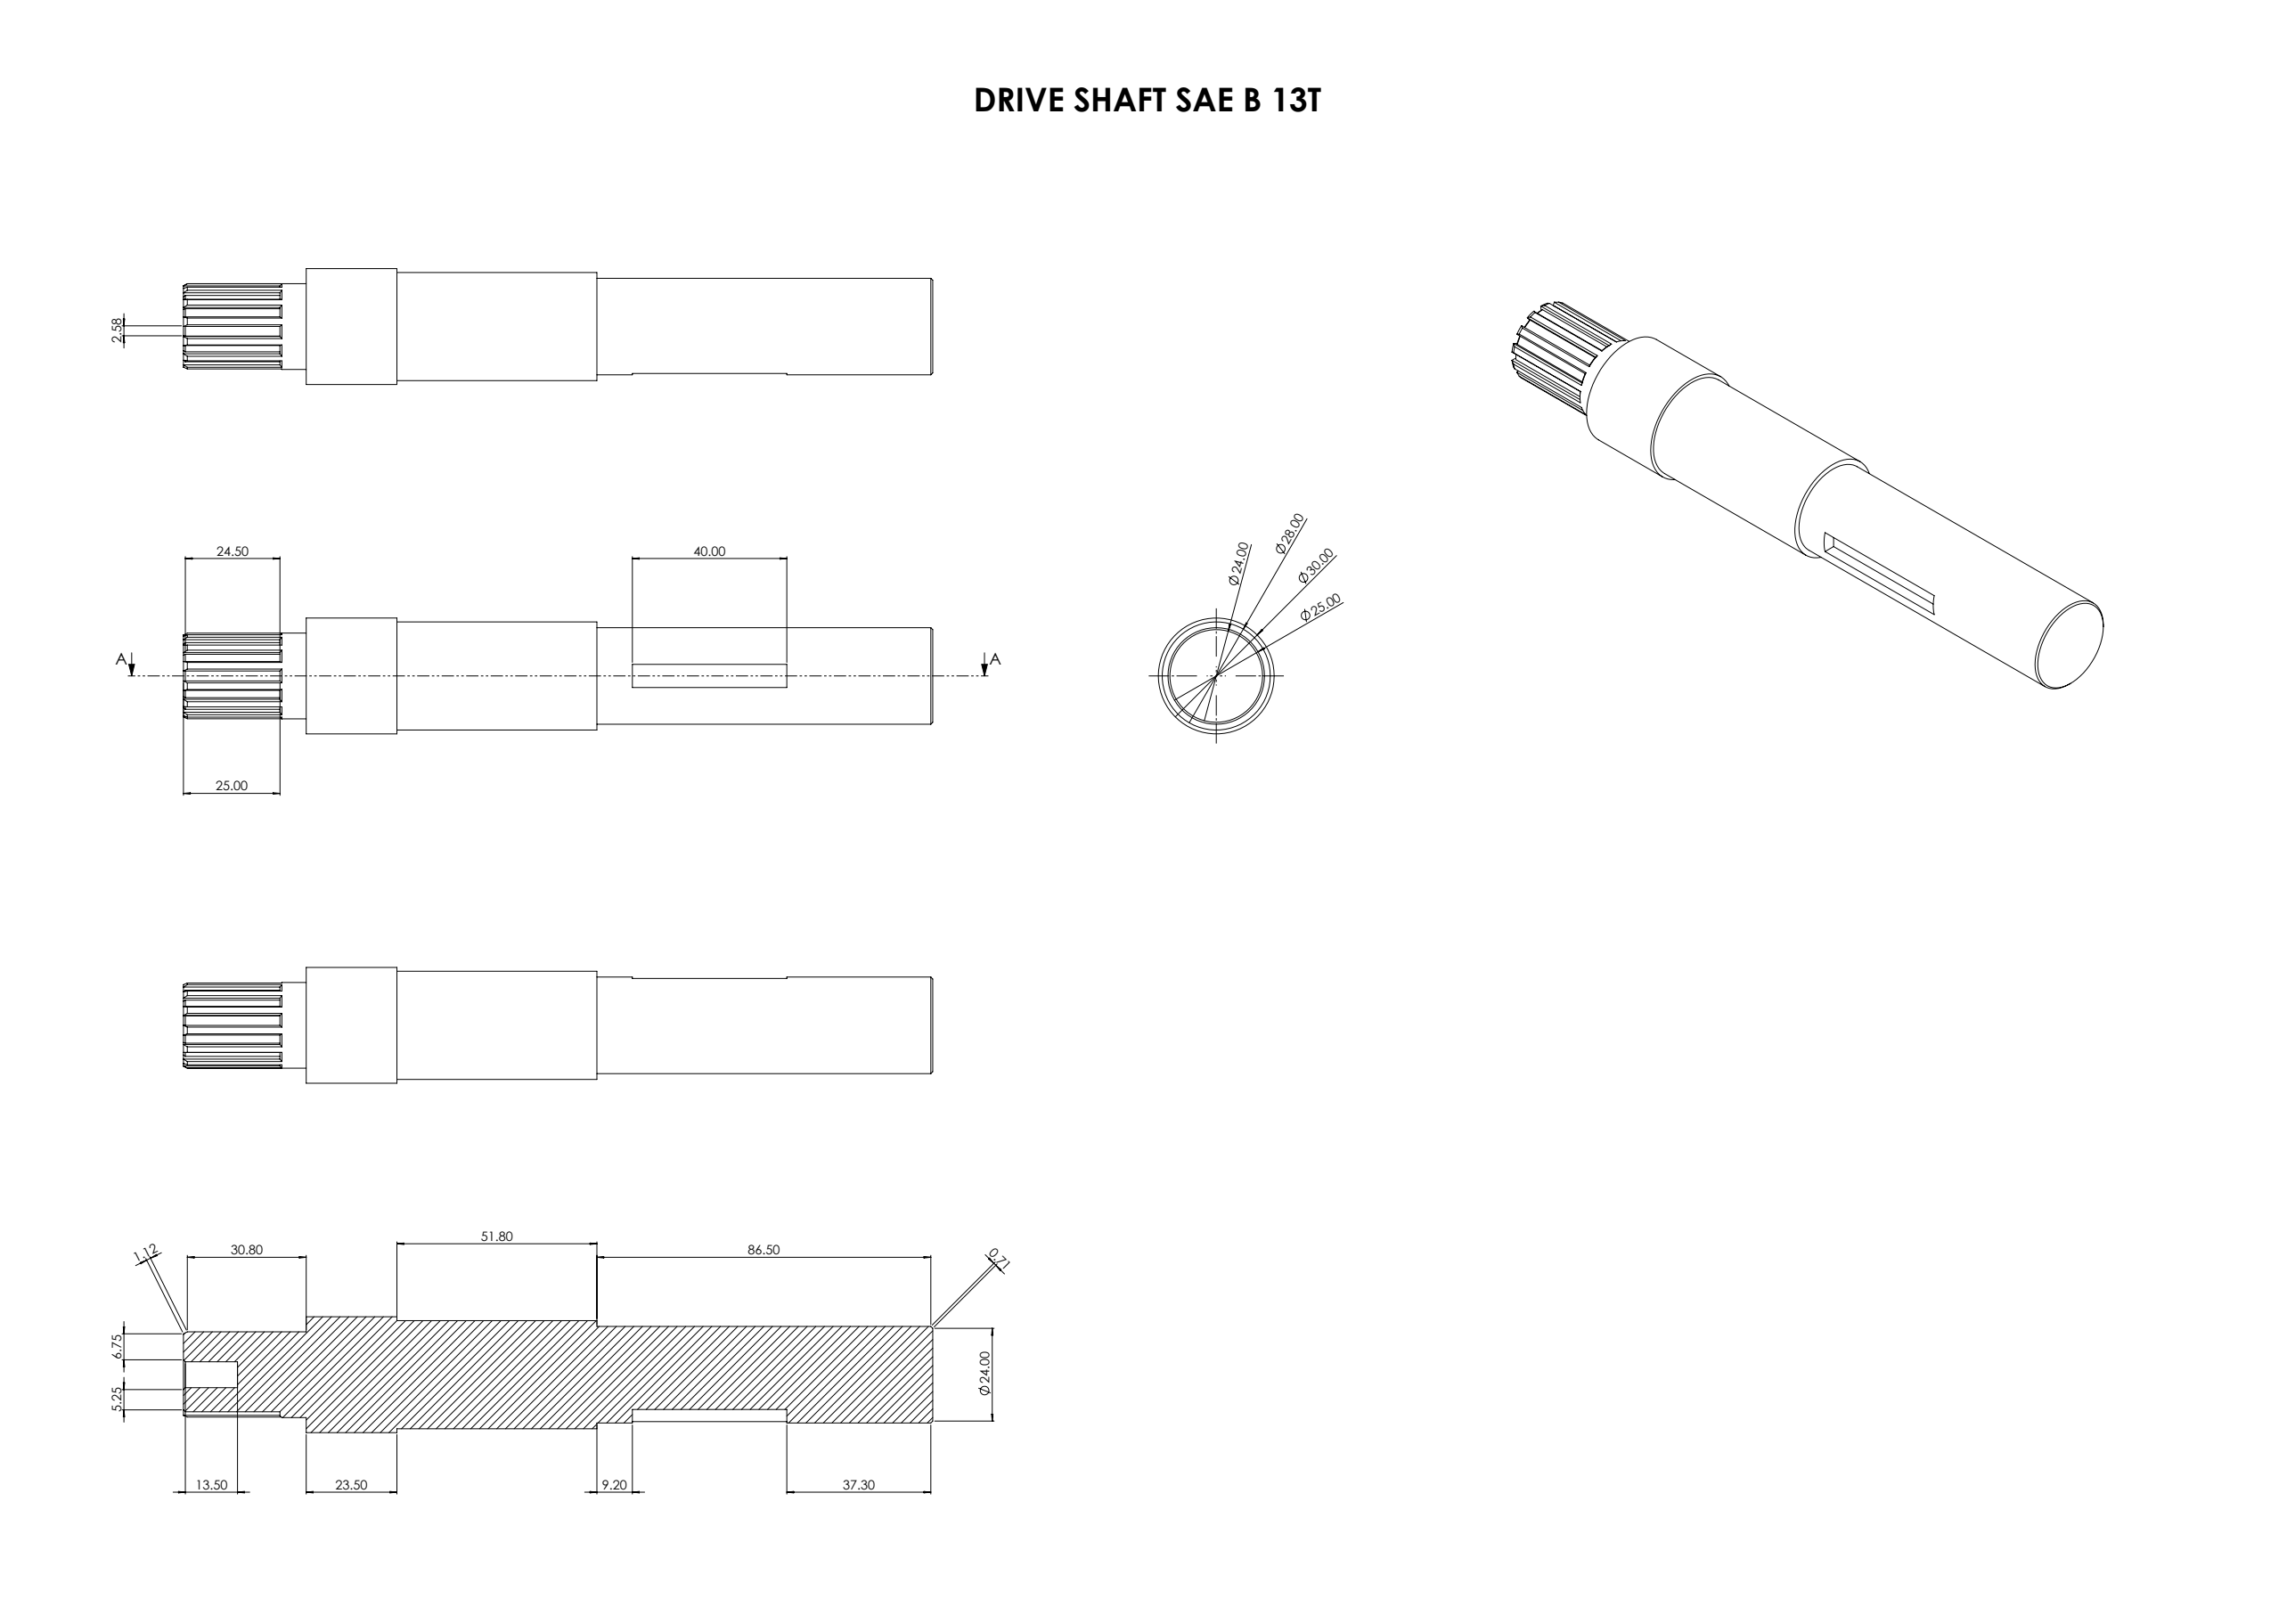
ISO-10303-21;
HEADER;
/* Generated by software containing ST-Developer
 * from STEP Tools, Inc. (www.steptools.com) 
 */

FILE_DESCRIPTION(
/* description */ (''),
/* implementation_level */ '2;1');

FILE_NAME(
/* name */ '09_Drive_Shaft_SAE_B_13T.step',
/* time_stamp */ '2026-10-26T07:49:00-07:00',
/* author */ (''),
/* organization */ (''),
/* preprocessor_version */ 'ST-DEVELOPER v20.2',
/* originating_system */ 'Autodesk Translation Framework v15.15.0.0',
/* authorisation */ '');

FILE_SCHEMA (('AUTOMOTIVE_DESIGN { 1 0 10303 214 3 1 1 }'));
ENDSEC;

DATA;
#10=MECHANICAL_DESIGN_GEOMETRIC_PRESENTATION_REPRESENTATION('',(#182),#38507);
#152=SHAPE_REPRESENTATION_RELATIONSHIP('SRR','None',#38580,#167);
#167=ADVANCED_BREP_SHAPE_REPRESENTATION('',(#197),#38497);
#182=STYLED_ITEM('',(#38720),#197);
#197=MANIFOLD_SOLID_BREP('Body1',#15076);
#338=(
BOUNDED_CURVE()
B_SPLINE_CURVE(2,(#25747,#25748,#25749),.UNSPECIFIED.,.F.,.F.)
B_SPLINE_CURVE_WITH_KNOTS((3,3),(0.00089915875038223,0.119861415155793),
 .UNSPECIFIED.)
CURVE()
GEOMETRIC_REPRESENTATION_ITEM()
RATIONAL_B_SPLINE_CURVE((1.00000690885838,1.00046048906391,1.))
REPRESENTATION_ITEM('')
);
#339=(
BOUNDED_CURVE()
B_SPLINE_CURVE(2,(#25761,#25762,#25763),.UNSPECIFIED.,.F.,.F.)
B_SPLINE_CURVE_WITH_KNOTS((3,3),(0.,0.118962256406331),.UNSPECIFIED.)
CURVE()
GEOMETRIC_REPRESENTATION_ITEM()
RATIONAL_B_SPLINE_CURVE((1.,1.00046048906569,1.0000069088584))
REPRESENTATION_ITEM('')
);
#340=(
BOUNDED_CURVE()
B_SPLINE_CURVE(2,(#25773,#25774,#25775),.UNSPECIFIED.,.F.,.F.)
B_SPLINE_CURVE_WITH_KNOTS((3,3),(-47.8696729569845,-47.8687190848821),
 .UNSPECIFIED.)
CURVE()
GEOMETRIC_REPRESENTATION_ITEM()
RATIONAL_B_SPLINE_CURVE((15.2054806811783,15.2077824060813,15.2100840336135))
REPRESENTATION_ITEM('')
);
#341=(
BOUNDED_CURVE()
B_SPLINE_CURVE(2,(#25778,#25779,#25780),.UNSPECIFIED.,.F.,.F.)
B_SPLINE_CURVE_WITH_KNOTS((3,3),(-2.77393487400909,-2.77298100190668),
 .UNSPECIFIED.)
CURVE()
GEOMETRIC_REPRESENTATION_ITEM()
RATIONAL_B_SPLINE_CURVE((15.2100840336134,15.2077824060812,15.2054806811782))
REPRESENTATION_ITEM('')
);
#342=(
BOUNDED_CURVE()
B_SPLINE_CURVE(2,(#25790,#25791,#25792),.UNSPECIFIED.,.F.,.F.)
B_SPLINE_CURVE_WITH_KNOTS((3,3),(0.111140514111159,0.111966209987666),
 .UNSPECIFIED.)
CURVE()
GEOMETRIC_REPRESENTATION_ITEM()
RATIONAL_B_SPLINE_CURVE((1.00000394455129,1.00000198692827,1.))
REPRESENTATION_ITEM('')
);
#343=(
BOUNDED_CURVE()
B_SPLINE_CURVE(2,(#25799,#25800,#25801),.UNSPECIFIED.,.F.,.F.)
B_SPLINE_CURVE_WITH_KNOTS((3,3),(0.,0.000825695876467816),.UNSPECIFIED.)
CURVE()
GEOMETRIC_REPRESENTATION_ITEM()
RATIONAL_B_SPLINE_CURVE((1.,1.00000198692868,1.00000394455211))
REPRESENTATION_ITEM('')
);
#344=(
BOUNDED_CURVE()
B_SPLINE_CURVE(2,(#25812,#25813,#25814),.UNSPECIFIED.,.F.,.F.)
B_SPLINE_CURVE_WITH_KNOTS((3,3),(0.000899158750379295,0.119861415155793),
 .UNSPECIFIED.)
CURVE()
GEOMETRIC_REPRESENTATION_ITEM()
RATIONAL_B_SPLINE_CURVE((1.00000690885842,1.00046048906656,1.))
REPRESENTATION_ITEM('')
);
#345=(
BOUNDED_CURVE()
B_SPLINE_CURVE(2,(#25826,#25827,#25828),.UNSPECIFIED.,.F.,.F.)
B_SPLINE_CURVE_WITH_KNOTS((3,3),(0.,0.11896225640633),.UNSPECIFIED.)
CURVE()
GEOMETRIC_REPRESENTATION_ITEM()
RATIONAL_B_SPLINE_CURVE((1.,1.00046048906395,1.00000690885837))
REPRESENTATION_ITEM('')
);
#346=(
BOUNDED_CURVE()
B_SPLINE_CURVE(2,(#25838,#25839,#25840),.UNSPECIFIED.,.F.,.F.)
B_SPLINE_CURVE_WITH_KNOTS((3,3),(-47.8696729569843,-47.8687190848819),
 .UNSPECIFIED.)
CURVE()
GEOMETRIC_REPRESENTATION_ITEM()
RATIONAL_B_SPLINE_CURVE((15.2054806811781,15.2077824060811,15.2100840336132))
REPRESENTATION_ITEM('')
);
#347=(
BOUNDED_CURVE()
B_SPLINE_CURVE(2,(#25843,#25844,#25845),.UNSPECIFIED.,.F.,.F.)
B_SPLINE_CURVE_WITH_KNOTS((3,3),(-2.77393487400938,-2.77298100190697),
 .UNSPECIFIED.)
CURVE()
GEOMETRIC_REPRESENTATION_ITEM()
RATIONAL_B_SPLINE_CURVE((15.2100840336132,15.2077824060811,15.2054806811781))
REPRESENTATION_ITEM('')
);
#348=(
BOUNDED_CURVE()
B_SPLINE_CURVE(2,(#25855,#25856,#25857),.UNSPECIFIED.,.F.,.F.)
B_SPLINE_CURVE_WITH_KNOTS((3,3),(0.111140514109634,0.111966209987666),
 .UNSPECIFIED.)
CURVE()
GEOMETRIC_REPRESENTATION_ITEM()
RATIONAL_B_SPLINE_CURVE((1.00000394455479,1.00000198693003,1.))
REPRESENTATION_ITEM('')
);
#349=(
BOUNDED_CURVE()
B_SPLINE_CURVE(2,(#25864,#25865,#25866),.UNSPECIFIED.,.F.,.F.)
B_SPLINE_CURVE_WITH_KNOTS((3,3),(0.,0.000825695875370319),.UNSPECIFIED.)
CURVE()
GEOMETRIC_REPRESENTATION_ITEM()
RATIONAL_B_SPLINE_CURVE((1.,1.00000198692765,1.00000394455006))
REPRESENTATION_ITEM('')
);
#350=(
BOUNDED_CURVE()
B_SPLINE_CURVE(2,(#25877,#25878,#25879),.UNSPECIFIED.,.F.,.F.)
B_SPLINE_CURVE_WITH_KNOTS((3,3),(0.000899158750382334,0.119861415155793),
 .UNSPECIFIED.)
CURVE()
GEOMETRIC_REPRESENTATION_ITEM()
RATIONAL_B_SPLINE_CURVE((1.00000690885837,1.00046048906313,1.))
REPRESENTATION_ITEM('')
);
#351=(
BOUNDED_CURVE()
B_SPLINE_CURVE(2,(#25891,#25892,#25893),.UNSPECIFIED.,.F.,.F.)
B_SPLINE_CURVE_WITH_KNOTS((3,3),(0.,0.11896225640633),.UNSPECIFIED.)
CURVE()
GEOMETRIC_REPRESENTATION_ITEM()
RATIONAL_B_SPLINE_CURVE((1.,1.00046048906413,1.00000690885838))
REPRESENTATION_ITEM('')
);
#352=(
BOUNDED_CURVE()
B_SPLINE_CURVE(2,(#25903,#25904,#25905),.UNSPECIFIED.,.F.,.F.)
B_SPLINE_CURVE_WITH_KNOTS((3,3),(-47.8696729569845,-47.8687190848821),
 .UNSPECIFIED.)
CURVE()
GEOMETRIC_REPRESENTATION_ITEM()
RATIONAL_B_SPLINE_CURVE((15.2054806811782,15.2077824060812,15.2100840336134))
REPRESENTATION_ITEM('')
);
#353=(
BOUNDED_CURVE()
B_SPLINE_CURVE(2,(#25908,#25909,#25910),.UNSPECIFIED.,.F.,.F.)
B_SPLINE_CURVE_WITH_KNOTS((3,3),(-2.77393487400914,-2.77298100190673),
 .UNSPECIFIED.)
CURVE()
GEOMETRIC_REPRESENTATION_ITEM()
RATIONAL_B_SPLINE_CURVE((15.2100840336134,15.2077824060812,15.2054806811782))
REPRESENTATION_ITEM('')
);
#354=(
BOUNDED_CURVE()
B_SPLINE_CURVE(2,(#25920,#25921,#25922),.UNSPECIFIED.,.F.,.F.)
B_SPLINE_CURVE_WITH_KNOTS((3,3),(0.111140514110888,0.111966209987666),
 .UNSPECIFIED.)
CURVE()
GEOMETRIC_REPRESENTATION_ITEM()
RATIONAL_B_SPLINE_CURVE((1.000003944553,1.00000198692913,1.))
REPRESENTATION_ITEM('')
);
#355=(
BOUNDED_CURVE()
B_SPLINE_CURVE(2,(#25929,#25930,#25931),.UNSPECIFIED.,.F.,.F.)
B_SPLINE_CURVE_WITH_KNOTS((3,3),(0.,0.000825695876921701),.UNSPECIFIED.)
CURVE()
GEOMETRIC_REPRESENTATION_ITEM()
RATIONAL_B_SPLINE_CURVE((1.,1.0000019869287,1.00000394455216))
REPRESENTATION_ITEM('')
);
#356=(
BOUNDED_CURVE()
B_SPLINE_CURVE(2,(#25942,#25943,#25944),.UNSPECIFIED.,.F.,.F.)
B_SPLINE_CURVE_WITH_KNOTS((3,3),(0.000899158750381089,0.119861415155793),
 .UNSPECIFIED.)
CURVE()
GEOMETRIC_REPRESENTATION_ITEM()
RATIONAL_B_SPLINE_CURVE((1.00000690885838,1.00046048906409,1.))
REPRESENTATION_ITEM('')
);
#357=(
BOUNDED_CURVE()
B_SPLINE_CURVE(2,(#25956,#25957,#25958),.UNSPECIFIED.,.F.,.F.)
B_SPLINE_CURVE_WITH_KNOTS((3,3),(0.,0.118962256406332),.UNSPECIFIED.)
CURVE()
GEOMETRIC_REPRESENTATION_ITEM()
RATIONAL_B_SPLINE_CURVE((1.,1.00046048906654,1.00000690885841))
REPRESENTATION_ITEM('')
);
#358=(
BOUNDED_CURVE()
B_SPLINE_CURVE(2,(#25968,#25969,#25970),.UNSPECIFIED.,.F.,.F.)
B_SPLINE_CURVE_WITH_KNOTS((3,3),(-47.8696729569844,-47.868719084882),
 .UNSPECIFIED.)
CURVE()
GEOMETRIC_REPRESENTATION_ITEM()
RATIONAL_B_SPLINE_CURVE((15.2054806811782,15.2077824060812,15.2100840336134))
REPRESENTATION_ITEM('')
);
#359=(
BOUNDED_CURVE()
B_SPLINE_CURVE(2,(#25973,#25974,#25975),.UNSPECIFIED.,.F.,.F.)
B_SPLINE_CURVE_WITH_KNOTS((3,3),(-2.77393487400941,-2.772981001907),
 .UNSPECIFIED.)
CURVE()
GEOMETRIC_REPRESENTATION_ITEM()
RATIONAL_B_SPLINE_CURVE((15.2100840336131,15.207782406081,15.205480681178))
REPRESENTATION_ITEM('')
);
#360=(
BOUNDED_CURVE()
B_SPLINE_CURVE(2,(#25985,#25986,#25987),.UNSPECIFIED.,.F.,.F.)
B_SPLINE_CURVE_WITH_KNOTS((3,3),(0.111140514110977,0.111966209987666),
 .UNSPECIFIED.)
CURVE()
GEOMETRIC_REPRESENTATION_ITEM()
RATIONAL_B_SPLINE_CURVE((1.00000394455159,1.00000198692842,1.))
REPRESENTATION_ITEM('')
);
#361=(
BOUNDED_CURVE()
B_SPLINE_CURVE(2,(#25994,#25995,#25996),.UNSPECIFIED.,.F.,.F.)
B_SPLINE_CURVE_WITH_KNOTS((3,3),(0.,0.000825695874631881),.UNSPECIFIED.)
CURVE()
GEOMETRIC_REPRESENTATION_ITEM()
RATIONAL_B_SPLINE_CURVE((1.,1.00000198692687,1.00000394454852))
REPRESENTATION_ITEM('')
);
#362=(
BOUNDED_CURVE()
B_SPLINE_CURVE(2,(#26005,#26006,#26007),.UNSPECIFIED.,.F.,.F.)
B_SPLINE_CURVE_WITH_KNOTS((3,3),(0.000899158750383316,0.119861415155793),
 .UNSPECIFIED.)
CURVE()
GEOMETRIC_REPRESENTATION_ITEM()
RATIONAL_B_SPLINE_CURVE((1.00000690885837,1.00046048906313,1.))
REPRESENTATION_ITEM('')
);
#363=(
BOUNDED_CURVE()
B_SPLINE_CURVE(2,(#26011,#26012,#26013),.UNSPECIFIED.,.F.,.F.)
B_SPLINE_CURVE_WITH_KNOTS((3,3),(1.83887863060053,1.88690815084928),
 .UNSPECIFIED.)
CURVE()
GEOMETRIC_REPRESENTATION_ITEM()
RATIONAL_B_SPLINE_CURVE((1.02805437145288,1.01439356064084,1.))
REPRESENTATION_ITEM('')
);
#364=(
BOUNDED_CURVE()
B_SPLINE_CURVE(2,(#26017,#26018,#26019),.UNSPECIFIED.,.F.,.F.)
B_SPLINE_CURVE_WITH_KNOTS((3,3),(0.0704444719086716,0.0709678248042913),
 .UNSPECIFIED.)
CURVE()
GEOMETRIC_REPRESENTATION_ITEM()
RATIONAL_B_SPLINE_CURVE((1.00000394455158,1.00000198692841,1.))
REPRESENTATION_ITEM('')
);
#365=(
BOUNDED_CURVE()
B_SPLINE_CURVE(2,(#26028,#26029,#26030),.UNSPECIFIED.,.F.,.F.)
B_SPLINE_CURVE_WITH_KNOTS((3,3),(0.111140514109306,0.111966209987666),
 .UNSPECIFIED.)
CURVE()
GEOMETRIC_REPRESENTATION_ITEM()
RATIONAL_B_SPLINE_CURVE((1.00000394455327,1.00000198692926,1.))
REPRESENTATION_ITEM('')
);
#366=(
BOUNDED_CURVE()
B_SPLINE_CURVE(2,(#26036,#26037,#26038),.UNSPECIFIED.,.F.,.F.)
B_SPLINE_CURVE_WITH_KNOTS((3,3),(0.,0.118962256406332),.UNSPECIFIED.)
CURVE()
GEOMETRIC_REPRESENTATION_ITEM()
RATIONAL_B_SPLINE_CURVE((1.,1.00046048906504,1.00000690885839))
REPRESENTATION_ITEM('')
);
#367=(
BOUNDED_CURVE()
B_SPLINE_CURVE(2,(#26049,#26050,#26051),.UNSPECIFIED.,.F.,.F.)
B_SPLINE_CURVE_WITH_KNOTS((3,3),(-47.8696729569846,-47.8687190848822),
 .UNSPECIFIED.)
CURVE()
GEOMETRIC_REPRESENTATION_ITEM()
RATIONAL_B_SPLINE_CURVE((15.2054806811784,15.2077824060813,15.2100840336135))
REPRESENTATION_ITEM('')
);
#368=(
BOUNDED_CURVE()
B_SPLINE_CURVE(2,(#26054,#26055,#26056),.UNSPECIFIED.,.F.,.F.)
B_SPLINE_CURVE_WITH_KNOTS((3,3),(0.,0.000825695876215709),.UNSPECIFIED.)
CURVE()
GEOMETRIC_REPRESENTATION_ITEM()
RATIONAL_B_SPLINE_CURVE((1.,1.00000198692775,1.00000394455027))
REPRESENTATION_ITEM('')
);
#369=(
BOUNDED_CURVE()
B_SPLINE_CURVE(2,(#26068,#26069,#26070),.UNSPECIFIED.,.F.,.F.)
B_SPLINE_CURVE_WITH_KNOTS((3,3),(0.000899158750381245,0.119861415155792),
 .UNSPECIFIED.)
CURVE()
GEOMETRIC_REPRESENTATION_ITEM()
RATIONAL_B_SPLINE_CURVE((1.00000690885837,1.00046048906334,1.))
REPRESENTATION_ITEM('')
);
#370=(
BOUNDED_CURVE()
B_SPLINE_CURVE(2,(#26072,#26073,#26074),.UNSPECIFIED.,.F.,.F.)
B_SPLINE_CURVE_WITH_KNOTS((3,3),(0.111140514111096,0.111966209987666),
 .UNSPECIFIED.)
CURVE()
GEOMETRIC_REPRESENTATION_ITEM()
RATIONAL_B_SPLINE_CURVE((1.00000394455331,1.00000198692928,1.))
REPRESENTATION_ITEM('')
);
#371=(
BOUNDED_CURVE()
B_SPLINE_CURVE(2,(#26158,#26159,#26160),.UNSPECIFIED.,.F.,.F.)
B_SPLINE_CURVE_WITH_KNOTS((3,3),(0.,0.118962256406332),.UNSPECIFIED.)
CURVE()
GEOMETRIC_REPRESENTATION_ITEM()
RATIONAL_B_SPLINE_CURVE((1.,1.00046048906488,1.00000690885839))
REPRESENTATION_ITEM('')
);
#372=(
BOUNDED_CURVE()
B_SPLINE_CURVE(2,(#26169,#26170,#26171),.UNSPECIFIED.,.F.,.F.)
B_SPLINE_CURVE_WITH_KNOTS((3,3),(-47.8696729569843,-47.8687190848819),
 .UNSPECIFIED.)
CURVE()
GEOMETRIC_REPRESENTATION_ITEM()
RATIONAL_B_SPLINE_CURVE((15.2054806811781,15.2077824060811,15.2100840336132))
REPRESENTATION_ITEM('')
);
#373=(
BOUNDED_CURVE()
B_SPLINE_CURVE(2,(#26174,#26175,#26176),.UNSPECIFIED.,.F.,.F.)
B_SPLINE_CURVE_WITH_KNOTS((3,3),(-2.77393487400923,-2.77298100190682),
 .UNSPECIFIED.)
CURVE()
GEOMETRIC_REPRESENTATION_ITEM()
RATIONAL_B_SPLINE_CURVE((15.2100840336133,15.2077824060812,15.2054806811782))
REPRESENTATION_ITEM('')
);
#374=(
BOUNDED_CURVE()
B_SPLINE_CURVE(2,(#26191,#26192,#26193),.UNSPECIFIED.,.F.,.F.)
B_SPLINE_CURVE_WITH_KNOTS((3,3),(0.,0.0008256958761486),.UNSPECIFIED.)
CURVE()
GEOMETRIC_REPRESENTATION_ITEM()
RATIONAL_B_SPLINE_CURVE((1.,1.00000198692878,1.00000394455231))
REPRESENTATION_ITEM('')
);
#375=(
BOUNDED_CURVE()
B_SPLINE_CURVE(2,(#26203,#26204,#26205),.UNSPECIFIED.,.F.,.F.)
B_SPLINE_CURVE_WITH_KNOTS((3,3),(0.000899158750380169,0.119861415155792),
 .UNSPECIFIED.)
CURVE()
GEOMETRIC_REPRESENTATION_ITEM()
RATIONAL_B_SPLINE_CURVE((1.0000069088584,1.00046048906499,1.))
REPRESENTATION_ITEM('')
);
#376=(
BOUNDED_CURVE()
B_SPLINE_CURVE(2,(#26212,#26213,#26214),.UNSPECIFIED.,.F.,.F.)
B_SPLINE_CURVE_WITH_KNOTS((3,3),(0.,0.118962256406331),.UNSPECIFIED.)
CURVE()
GEOMETRIC_REPRESENTATION_ITEM()
RATIONAL_B_SPLINE_CURVE((1.,1.00046048906418,1.00000690885838))
REPRESENTATION_ITEM('')
);
#377=(
BOUNDED_CURVE()
B_SPLINE_CURVE(2,(#26223,#26224,#26225),.UNSPECIFIED.,.F.,.F.)
B_SPLINE_CURVE_WITH_KNOTS((3,3),(-47.8696729569847,-47.8687190848823),
 .UNSPECIFIED.)
CURVE()
GEOMETRIC_REPRESENTATION_ITEM()
RATIONAL_B_SPLINE_CURVE((15.2054806811785,15.2077824060814,15.2100840336136))
REPRESENTATION_ITEM('')
);
#378=(
BOUNDED_CURVE()
B_SPLINE_CURVE(2,(#26228,#26229,#26230),.UNSPECIFIED.,.F.,.F.)
B_SPLINE_CURVE_WITH_KNOTS((3,3),(-2.77393487400886,-2.77298100190645),
 .UNSPECIFIED.)
CURVE()
GEOMETRIC_REPRESENTATION_ITEM()
RATIONAL_B_SPLINE_CURVE((15.2100840336136,15.2077824060815,15.2054806811785))
REPRESENTATION_ITEM('')
);
#379=(
BOUNDED_CURVE()
B_SPLINE_CURVE(2,(#26240,#26241,#26242),.UNSPECIFIED.,.F.,.F.)
B_SPLINE_CURVE_WITH_KNOTS((3,3),(0.111140514112235,0.111966209987666),
 .UNSPECIFIED.)
CURVE()
GEOMETRIC_REPRESENTATION_ITEM()
RATIONAL_B_SPLINE_CURVE((1.00000394455079,1.00000198692802,1.))
REPRESENTATION_ITEM('')
);
#380=(
BOUNDED_CURVE()
B_SPLINE_CURVE(2,(#26249,#26250,#26251),.UNSPECIFIED.,.F.,.F.)
B_SPLINE_CURVE_WITH_KNOTS((3,3),(0.,0.000825695876969575),.UNSPECIFIED.)
CURVE()
GEOMETRIC_REPRESENTATION_ITEM()
RATIONAL_B_SPLINE_CURVE((1.,1.00000198692876,1.00000394455228))
REPRESENTATION_ITEM('')
);
#381=(
BOUNDED_CURVE()
B_SPLINE_CURVE(2,(#26365,#26366,#26367),.UNSPECIFIED.,.F.,.F.)
B_SPLINE_CURVE_WITH_KNOTS((3,3),(0.000899158750381918,0.119861415155793),
 .UNSPECIFIED.)
CURVE()
GEOMETRIC_REPRESENTATION_ITEM()
RATIONAL_B_SPLINE_CURVE((1.00000690885838,1.00046048906396,1.))
REPRESENTATION_ITEM('')
);
#382=(
BOUNDED_CURVE()
B_SPLINE_CURVE(2,(#26374,#26375,#26376),.UNSPECIFIED.,.F.,.F.)
B_SPLINE_CURVE_WITH_KNOTS((3,3),(0.,0.118962256406328),.UNSPECIFIED.)
CURVE()
GEOMETRIC_REPRESENTATION_ITEM()
RATIONAL_B_SPLINE_CURVE((1.,1.00046048906152,1.00000690885834))
REPRESENTATION_ITEM('')
);
#383=(
BOUNDED_CURVE()
B_SPLINE_CURVE(2,(#26385,#26386,#26387),.UNSPECIFIED.,.F.,.F.)
B_SPLINE_CURVE_WITH_KNOTS((3,3),(-47.8696729569843,-47.8687190848818),
 .UNSPECIFIED.)
CURVE()
GEOMETRIC_REPRESENTATION_ITEM()
RATIONAL_B_SPLINE_CURVE((15.2054806811781,15.207782406081,15.2100840336132))
REPRESENTATION_ITEM('')
);
#384=(
BOUNDED_CURVE()
B_SPLINE_CURVE(2,(#26390,#26391,#26392),.UNSPECIFIED.,.F.,.F.)
B_SPLINE_CURVE_WITH_KNOTS((3,3),(-2.7739348740092,-2.77298100190679),
 .UNSPECIFIED.)
CURVE()
GEOMETRIC_REPRESENTATION_ITEM()
RATIONAL_B_SPLINE_CURVE((15.2100840336132,15.2077824060811,15.2054806811781))
REPRESENTATION_ITEM('')
);
#385=(
BOUNDED_CURVE()
B_SPLINE_CURVE(2,(#26397,#26398,#26399),.UNSPECIFIED.,.F.,.F.)
B_SPLINE_CURVE_WITH_KNOTS((3,3),(0.111140514111405,0.111966209987666),
 .UNSPECIFIED.)
CURVE()
GEOMETRIC_REPRESENTATION_ITEM()
RATIONAL_B_SPLINE_CURVE((1.00000394455238,1.00000198692881,1.))
REPRESENTATION_ITEM('')
);
#386=(
BOUNDED_CURVE()
B_SPLINE_CURVE(2,(#26404,#26405,#26406),.UNSPECIFIED.,.F.,.F.)
B_SPLINE_CURVE_WITH_KNOTS((3,3),(0.,0.000825695877819724),.UNSPECIFIED.)
CURVE()
GEOMETRIC_REPRESENTATION_ITEM()
RATIONAL_B_SPLINE_CURVE((1.,1.00000198693025,1.00000394455522))
REPRESENTATION_ITEM('')
);
#387=(
BOUNDED_CURVE()
B_SPLINE_CURVE(2,(#26412,#26413,#26414),.UNSPECIFIED.,.F.,.F.)
B_SPLINE_CURVE_WITH_KNOTS((3,3),(0.000899158750380705,0.119861415155793),
 .UNSPECIFIED.)
CURVE()
GEOMETRIC_REPRESENTATION_ITEM()
RATIONAL_B_SPLINE_CURVE((1.00000690885837,1.0004604890632,1.))
REPRESENTATION_ITEM('')
);
#388=(
BOUNDED_CURVE()
B_SPLINE_CURVE(2,(#26421,#26422,#26423),.UNSPECIFIED.,.F.,.F.)
B_SPLINE_CURVE_WITH_KNOTS((3,3),(0.,0.118962256406331),.UNSPECIFIED.)
CURVE()
GEOMETRIC_REPRESENTATION_ITEM()
RATIONAL_B_SPLINE_CURVE((1.,1.00046048906486,1.00000690885839))
REPRESENTATION_ITEM('')
);
#389=(
BOUNDED_CURVE()
B_SPLINE_CURVE(2,(#26432,#26433,#26434),.UNSPECIFIED.,.F.,.F.)
B_SPLINE_CURVE_WITH_KNOTS((3,3),(-47.8696729569845,-47.8687190848821),
 .UNSPECIFIED.)
CURVE()
GEOMETRIC_REPRESENTATION_ITEM()
RATIONAL_B_SPLINE_CURVE((15.2054806811783,15.2077824060812,15.2100840336134))
REPRESENTATION_ITEM('')
);
#390=(
BOUNDED_CURVE()
B_SPLINE_CURVE(2,(#26437,#26438,#26439),.UNSPECIFIED.,.F.,.F.)
B_SPLINE_CURVE_WITH_KNOTS((3,3),(-2.77393487400922,-2.77298100190681),
 .UNSPECIFIED.)
CURVE()
GEOMETRIC_REPRESENTATION_ITEM()
RATIONAL_B_SPLINE_CURVE((15.2100840336133,15.2077824060812,15.2054806811782))
REPRESENTATION_ITEM('')
);
#391=(
BOUNDED_CURVE()
B_SPLINE_CURVE(2,(#26444,#26445,#26446),.UNSPECIFIED.,.F.,.F.)
B_SPLINE_CURVE_WITH_KNOTS((3,3),(0.111140514110649,0.111966209987666),
 .UNSPECIFIED.)
CURVE()
GEOMETRIC_REPRESENTATION_ITEM()
RATIONAL_B_SPLINE_CURVE((1.00000394455082,1.00000198692803,1.))
REPRESENTATION_ITEM('')
);
#392=(
BOUNDED_CURVE()
B_SPLINE_CURVE(2,(#26451,#26452,#26453),.UNSPECIFIED.,.F.,.F.)
B_SPLINE_CURVE_WITH_KNOTS((3,3),(0.,0.000825695875329356),.UNSPECIFIED.)
CURVE()
GEOMETRIC_REPRESENTATION_ITEM()
RATIONAL_B_SPLINE_CURVE((1.,1.00000198692802,1.00000394455079))
REPRESENTATION_ITEM('')
);
#393=(
BOUNDED_CURVE()
B_SPLINE_CURVE(2,(#26459,#26460,#26461),.UNSPECIFIED.,.F.,.F.)
B_SPLINE_CURVE_WITH_KNOTS((3,3),(0.000899158750382631,0.119861415155793),
 .UNSPECIFIED.)
CURVE()
GEOMETRIC_REPRESENTATION_ITEM()
RATIONAL_B_SPLINE_CURVE((1.00000690885839,1.0004604890648,1.))
REPRESENTATION_ITEM('')
);
#394=(
BOUNDED_CURVE()
B_SPLINE_CURVE(2,(#26468,#26469,#26470),.UNSPECIFIED.,.F.,.F.)
B_SPLINE_CURVE_WITH_KNOTS((3,3),(0.,0.118962256406331),.UNSPECIFIED.)
CURVE()
GEOMETRIC_REPRESENTATION_ITEM()
RATIONAL_B_SPLINE_CURVE((1.,1.00046048906397,1.00000690885837))
REPRESENTATION_ITEM('')
);
#395=(
BOUNDED_CURVE()
B_SPLINE_CURVE(2,(#26479,#26480,#26481),.UNSPECIFIED.,.F.,.F.)
B_SPLINE_CURVE_WITH_KNOTS((3,3),(-47.8696729569844,-47.868719084882),
 .UNSPECIFIED.)
CURVE()
GEOMETRIC_REPRESENTATION_ITEM()
RATIONAL_B_SPLINE_CURVE((15.2054806811782,15.2077824060812,15.2100840336133))
REPRESENTATION_ITEM('')
);
#396=(
BOUNDED_CURVE()
B_SPLINE_CURVE(2,(#26484,#26485,#26486),.UNSPECIFIED.,.F.,.F.)
B_SPLINE_CURVE_WITH_KNOTS((3,3),(-2.77393487400938,-2.77298100190697),
 .UNSPECIFIED.)
CURVE()
GEOMETRIC_REPRESENTATION_ITEM()
RATIONAL_B_SPLINE_CURVE((15.2100840336132,15.207782406081,15.205480681178))
REPRESENTATION_ITEM('')
);
#397=(
BOUNDED_CURVE()
B_SPLINE_CURVE(2,(#26491,#26492,#26493),.UNSPECIFIED.,.F.,.F.)
B_SPLINE_CURVE_WITH_KNOTS((3,3),(0.111140514111592,0.111966209987666),
 .UNSPECIFIED.)
CURVE()
GEOMETRIC_REPRESENTATION_ITEM()
RATIONAL_B_SPLINE_CURVE((1.00000394455076,1.000001986928,1.))
REPRESENTATION_ITEM('')
);
#398=(
BOUNDED_CURVE()
B_SPLINE_CURVE(2,(#26498,#26499,#26500),.UNSPECIFIED.,.F.,.F.)
B_SPLINE_CURVE_WITH_KNOTS((3,3),(0.,0.00082569587425766),.UNSPECIFIED.)
CURVE()
GEOMETRIC_REPRESENTATION_ITEM()
RATIONAL_B_SPLINE_CURVE((1.,1.00000198692851,1.00000394455177))
REPRESENTATION_ITEM('')
);
#399=(
BOUNDED_CURVE()
B_SPLINE_CURVE(2,(#26506,#26507,#26508),.UNSPECIFIED.,.F.,.F.)
B_SPLINE_CURVE_WITH_KNOTS((3,3),(0.000899158750379694,0.119861415155793),
 .UNSPECIFIED.)
CURVE()
GEOMETRIC_REPRESENTATION_ITEM()
RATIONAL_B_SPLINE_CURVE((1.00000690885841,1.00046048906573,1.))
REPRESENTATION_ITEM('')
);
#400=(
BOUNDED_CURVE()
B_SPLINE_CURVE(2,(#26515,#26516,#26517),.UNSPECIFIED.,.F.,.F.)
B_SPLINE_CURVE_WITH_KNOTS((3,3),(0.,0.118962256406331),.UNSPECIFIED.)
CURVE()
GEOMETRIC_REPRESENTATION_ITEM()
RATIONAL_B_SPLINE_CURVE((1.,1.00046048906579,1.0000069088584))
REPRESENTATION_ITEM('')
);
#401=(
BOUNDED_CURVE()
B_SPLINE_CURVE(2,(#26526,#26527,#26528),.UNSPECIFIED.,.F.,.F.)
B_SPLINE_CURVE_WITH_KNOTS((3,3),(-47.8696729569842,-47.8687190848818),
 .UNSPECIFIED.)
CURVE()
GEOMETRIC_REPRESENTATION_ITEM()
RATIONAL_B_SPLINE_CURVE((15.205480681178,15.207782406081,15.2100840336131))
REPRESENTATION_ITEM('')
);
#402=(
BOUNDED_CURVE()
B_SPLINE_CURVE(2,(#26531,#26532,#26533),.UNSPECIFIED.,.F.,.F.)
B_SPLINE_CURVE_WITH_KNOTS((3,3),(-2.77393487400937,-2.77298100190696),
 .UNSPECIFIED.)
CURVE()
GEOMETRIC_REPRESENTATION_ITEM()
RATIONAL_B_SPLINE_CURVE((15.2100840336132,15.207782406081,15.205480681178))
REPRESENTATION_ITEM('')
);
#403=(
BOUNDED_CURVE()
B_SPLINE_CURVE(2,(#26538,#26539,#26540),.UNSPECIFIED.,.F.,.F.)
B_SPLINE_CURVE_WITH_KNOTS((3,3),(0.111140514111407,0.111966209987666),
 .UNSPECIFIED.)
CURVE()
GEOMETRIC_REPRESENTATION_ITEM()
RATIONAL_B_SPLINE_CURVE((1.00000394455114,1.00000198692819,1.))
REPRESENTATION_ITEM('')
);
#404=(
BOUNDED_CURVE()
B_SPLINE_CURVE(2,(#26545,#26546,#26547),.UNSPECIFIED.,.F.,.F.)
B_SPLINE_CURVE_WITH_KNOTS((3,3),(0.,0.000825695875568355),.UNSPECIFIED.)
CURVE()
GEOMETRIC_REPRESENTATION_ITEM()
RATIONAL_B_SPLINE_CURVE((1.,1.00000198692854,1.00000394455182))
REPRESENTATION_ITEM('')
);
#405=(
BOUNDED_CURVE()
B_SPLINE_CURVE(2,(#26553,#26554,#26555),.UNSPECIFIED.,.F.,.F.)
B_SPLINE_CURVE_WITH_KNOTS((3,3),(0.000899158750377779,0.119861415155792),
 .UNSPECIFIED.)
CURVE()
GEOMETRIC_REPRESENTATION_ITEM()
RATIONAL_B_SPLINE_CURVE((1.00000690885845,1.00046048906834,1.))
REPRESENTATION_ITEM('')
);
#406=(
BOUNDED_CURVE()
B_SPLINE_CURVE(2,(#26562,#26563,#26564),.UNSPECIFIED.,.F.,.F.)
B_SPLINE_CURVE_WITH_KNOTS((3,3),(0.,0.118962256406334),.UNSPECIFIED.)
CURVE()
GEOMETRIC_REPRESENTATION_ITEM()
RATIONAL_B_SPLINE_CURVE((1.,1.00046048906835,1.00000690885844))
REPRESENTATION_ITEM('')
);
#407=(
BOUNDED_CURVE()
B_SPLINE_CURVE(2,(#26573,#26574,#26575),.UNSPECIFIED.,.F.,.F.)
B_SPLINE_CURVE_WITH_KNOTS((3,3),(-47.8696729569843,-47.8687190848819),
 .UNSPECIFIED.)
CURVE()
GEOMETRIC_REPRESENTATION_ITEM()
RATIONAL_B_SPLINE_CURVE((15.2054806811781,15.2077824060811,15.2100840336133))
REPRESENTATION_ITEM('')
);
#408=(
BOUNDED_CURVE()
B_SPLINE_CURVE(2,(#26578,#26579,#26580),.UNSPECIFIED.,.F.,.F.)
B_SPLINE_CURVE_WITH_KNOTS((3,3),(-2.77393487400929,-2.77298100190688),
 .UNSPECIFIED.)
CURVE()
GEOMETRIC_REPRESENTATION_ITEM()
RATIONAL_B_SPLINE_CURVE((15.2100840336132,15.207782406081,15.205480681178))
REPRESENTATION_ITEM('')
);
#409=(
BOUNDED_CURVE()
B_SPLINE_CURVE(2,(#26586,#26587,#26588),.UNSPECIFIED.,.F.,.F.)
B_SPLINE_CURVE_WITH_KNOTS((3,3),(0.,0.000825695878712508),.UNSPECIFIED.)
CURVE()
GEOMETRIC_REPRESENTATION_ITEM()
RATIONAL_B_SPLINE_CURVE((1.,1.00000198693036,1.00000394455544))
REPRESENTATION_ITEM('')
);
#410=(
BOUNDED_CURVE()
B_SPLINE_CURVE(2,(#26592,#26593,#26594),.UNSPECIFIED.,.F.,.F.)
B_SPLINE_CURVE_WITH_KNOTS((3,3),(0.0008991587503824,0.119861415155793),
 .UNSPECIFIED.)
CURVE()
GEOMETRIC_REPRESENTATION_ITEM()
RATIONAL_B_SPLINE_CURVE((1.0000069088584,1.00046048906496,1.))
REPRESENTATION_ITEM('')
);
#411=(
BOUNDED_CURVE()
B_SPLINE_CURVE(2,(#26596,#26597,#26598),.UNSPECIFIED.,.F.,.F.)
B_SPLINE_CURVE_WITH_KNOTS((3,3),(0.111140514113447,0.111966209987666),
 .UNSPECIFIED.)
CURVE()
GEOMETRIC_REPRESENTATION_ITEM()
RATIONAL_B_SPLINE_CURVE((1.0000039445487,1.00000198692696,1.))
REPRESENTATION_ITEM('')
);
#412=(
BOUNDED_CURVE()
B_SPLINE_CURVE(2,(#26624,#26625,#26626),.UNSPECIFIED.,.F.,.F.)
B_SPLINE_CURVE_WITH_KNOTS((3,3),(0.,0.118962256406329),.UNSPECIFIED.)
CURVE()
GEOMETRIC_REPRESENTATION_ITEM()
RATIONAL_B_SPLINE_CURVE((1.,1.00046048906511,1.00000690885839))
REPRESENTATION_ITEM('')
);
#413=(
BOUNDED_CURVE()
B_SPLINE_CURVE(2,(#26635,#26636,#26637),.UNSPECIFIED.,.F.,.F.)
B_SPLINE_CURVE_WITH_KNOTS((3,3),(-47.8696729569844,-47.868719084882),
 .UNSPECIFIED.)
CURVE()
GEOMETRIC_REPRESENTATION_ITEM()
RATIONAL_B_SPLINE_CURVE((15.2054806811782,15.2077824060812,15.2100840336133))
REPRESENTATION_ITEM('')
);
#414=(
BOUNDED_CURVE()
B_SPLINE_CURVE(2,(#26640,#26641,#26642),.UNSPECIFIED.,.F.,.F.)
B_SPLINE_CURVE_WITH_KNOTS((3,3),(-2.77393487400909,-2.77298100190668),
 .UNSPECIFIED.)
CURVE()
GEOMETRIC_REPRESENTATION_ITEM()
RATIONAL_B_SPLINE_CURVE((15.2100840336134,15.2077824060812,15.2054806811782))
REPRESENTATION_ITEM('')
);
#415=(
BOUNDED_CURVE()
B_SPLINE_CURVE(2,(#26648,#26649,#26650),.UNSPECIFIED.,.F.,.F.)
B_SPLINE_CURVE_WITH_KNOTS((3,3),(0.,0.000825695876243723),.UNSPECIFIED.)
CURVE()
GEOMETRIC_REPRESENTATION_ITEM()
RATIONAL_B_SPLINE_CURVE((1.,1.00000198692885,1.00000394455244))
REPRESENTATION_ITEM('')
);
#416=(
BOUNDED_CURVE()
B_SPLINE_CURVE(2,(#26716,#26717,#26718),.UNSPECIFIED.,.F.,.F.)
B_SPLINE_CURVE_WITH_KNOTS((3,3),(0.111140514108954,0.111966209987666),
 .UNSPECIFIED.)
CURVE()
GEOMETRIC_REPRESENTATION_ITEM()
RATIONAL_B_SPLINE_CURVE((1.00000394455544,1.00000198693036,1.))
REPRESENTATION_ITEM('')
);
#486=FACE_BOUND('',#3042,.T.);
#487=FACE_BOUND('',#3063,.T.);
#488=FACE_BOUND('',#3066,.T.);
#489=FACE_BOUND('',#3069,.T.);
#490=FACE_BOUND('',#3071,.T.);
#666=PLANE('',#15951);
#667=PLANE('',#15952);
#668=PLANE('',#15956);
#669=PLANE('',#15957);
#670=PLANE('',#15958);
#671=PLANE('',#15959);
#672=PLANE('',#15960);
#673=PLANE('',#15964);
#674=PLANE('',#15965);
#675=PLANE('',#15966);
#676=PLANE('',#15967);
#677=PLANE('',#15968);
#678=PLANE('',#15972);
#679=PLANE('',#15973);
#680=PLANE('',#15974);
#681=PLANE('',#15975);
#682=PLANE('',#15976);
#683=PLANE('',#15980);
#684=PLANE('',#15981);
#685=PLANE('',#15982);
#686=PLANE('',#15983);
#687=PLANE('',#15984);
#688=PLANE('',#15985);
#689=PLANE('',#15989);
#690=PLANE('',#16016);
#691=PLANE('',#16017);
#692=PLANE('',#16020);
#693=PLANE('',#16021);
#694=PLANE('',#16022);
#695=PLANE('',#16023);
#696=PLANE('',#16024);
#697=PLANE('',#16027);
#698=PLANE('',#16028);
#699=PLANE('',#16029);
#700=PLANE('',#16030);
#701=PLANE('',#16031);
#702=PLANE('',#16032);
#703=PLANE('',#16033);
#704=PLANE('',#16034);
#705=PLANE('',#16035);
#706=PLANE('',#16036);
#707=PLANE('',#16037);
#708=PLANE('',#16038);
#709=PLANE('',#16039);
#710=PLANE('',#16040);
#711=PLANE('',#16041);
#712=PLANE('',#16042);
#713=PLANE('',#16043);
#714=PLANE('',#16044);
#715=PLANE('',#16045);
#716=PLANE('',#16046);
#717=PLANE('',#16047);
#718=PLANE('',#16048);
#719=PLANE('',#16049);
#720=PLANE('',#16050);
#721=PLANE('',#16051);
#722=PLANE('',#16052);
#723=PLANE('',#16053);
#724=PLANE('',#16054);
#725=PLANE('',#16055);
#726=PLANE('',#16058);
#727=PLANE('',#16059);
#728=PLANE('',#16060);
#729=PLANE('',#16061);
#730=PLANE('',#16062);
#731=PLANE('',#16065);
#732=PLANE('',#16066);
#733=PLANE('',#16067);
#734=PLANE('',#16068);
#735=PLANE('',#16069);
#736=PLANE('',#16072);
#737=PLANE('',#16073);
#738=PLANE('',#16074);
#739=PLANE('',#16075);
#740=PLANE('',#16076);
#741=PLANE('',#16079);
#742=PLANE('',#16080);
#743=PLANE('',#16081);
#744=PLANE('',#16082);
#745=PLANE('',#16083);
#746=PLANE('',#16086);
#747=PLANE('',#16087);
#748=PLANE('',#16090);
#749=PLANE('',#16091);
#750=PLANE('',#16092);
#751=PLANE('',#16093);
#752=PLANE('',#16096);
#753=PLANE('',#16097);
#754=PLANE('',#16105);
#755=PLANE('',#16116);
#756=PLANE('',#16117);
#757=PLANE('',#16119);
#758=PLANE('',#16120);
#759=PLANE('',#16121);
#760=PLANE('',#16123);
#761=PLANE('',#16124);
#762=PLANE('',#16129);
#763=PLANE('',#16135);
#764=PLANE('',#16137);
#765=PLANE('',#16141);
#766=PLANE('',#16145);
#767=PLANE('',#16151);
#1162=B_SPLINE_CURVE_WITH_KNOTS('',3,(#25752,#25753,#25754,#25755),
 .UNSPECIFIED.,.F.,.F.,(4,4),(-0.082197241799306,0.),.UNSPECIFIED.);
#1163=B_SPLINE_CURVE_WITH_KNOTS('',3,(#25766,#25767,#25768,#25769),
 .UNSPECIFIED.,.F.,.F.,(4,4),(-0.0821909663426025,0.),.UNSPECIFIED.);
#1164=B_SPLINE_CURVE_WITH_KNOTS('',3,(#25817,#25818,#25819,#25820),
 .UNSPECIFIED.,.F.,.F.,(4,4),(-0.0821972417993003,0.),.UNSPECIFIED.);
#1165=B_SPLINE_CURVE_WITH_KNOTS('',3,(#25831,#25832,#25833,#25834),
 .UNSPECIFIED.,.F.,.F.,(4,4),(-0.0821909663425251,0.),.UNSPECIFIED.);
#1166=B_SPLINE_CURVE_WITH_KNOTS('',3,(#25882,#25883,#25884,#25885),
 .UNSPECIFIED.,.F.,.F.,(4,4),(-0.0821972417992908,0.),.UNSPECIFIED.);
#1167=B_SPLINE_CURVE_WITH_KNOTS('',3,(#25896,#25897,#25898,#25899),
 .UNSPECIFIED.,.F.,.F.,(4,4),(-0.0821909663425343,0.),.UNSPECIFIED.);
#1168=B_SPLINE_CURVE_WITH_KNOTS('',3,(#25947,#25948,#25949,#25950),
 .UNSPECIFIED.,.F.,.F.,(4,4),(-0.0821972417992827,0.),.UNSPECIFIED.);
#1169=B_SPLINE_CURVE_WITH_KNOTS('',3,(#25961,#25962,#25963,#25964),
 .UNSPECIFIED.,.F.,.F.,(4,4),(-0.0821909663425014,0.),.UNSPECIFIED.);
#1170=B_SPLINE_CURVE_WITH_KNOTS('',3,(#26041,#26042,#26043,#26044),
 .UNSPECIFIED.,.F.,.F.,(4,4),(-0.0821909663426067,0.),.UNSPECIFIED.);
#1171=B_SPLINE_CURVE_WITH_KNOTS('',3,(#26152,#26153,#26154,#26155),
 .UNSPECIFIED.,.F.,.F.,(4,4),(-0.0821972417992939,0.),.UNSPECIFIED.);
#1172=B_SPLINE_CURVE_WITH_KNOTS('',3,(#26163,#26164,#26165,#26166),
 .UNSPECIFIED.,.F.,.F.,(4,4),(-0.0821909663424864,0.),.UNSPECIFIED.);
#1173=B_SPLINE_CURVE_WITH_KNOTS('',3,(#26206,#26207,#26208,#26209),
 .UNSPECIFIED.,.F.,.F.,(4,4),(-0.0821972417992863,0.),.UNSPECIFIED.);
#1174=B_SPLINE_CURVE_WITH_KNOTS('',3,(#26217,#26218,#26219,#26220),
 .UNSPECIFIED.,.F.,.F.,(4,4),(-0.0821909663425319,0.),.UNSPECIFIED.);
#1175=B_SPLINE_CURVE_WITH_KNOTS('',3,(#26368,#26369,#26370,#26371),
 .UNSPECIFIED.,.F.,.F.,(4,4),(-0.0821972417993165,0.),.UNSPECIFIED.);
#1176=B_SPLINE_CURVE_WITH_KNOTS('',3,(#26379,#26380,#26381,#26382),
 .UNSPECIFIED.,.F.,.F.,(4,4),(-0.0821909663426151,0.),.UNSPECIFIED.);
#1177=B_SPLINE_CURVE_WITH_KNOTS('',3,(#26415,#26416,#26417,#26418),
 .UNSPECIFIED.,.F.,.F.,(4,4),(-0.0821972417992918,0.),.UNSPECIFIED.);
#1178=B_SPLINE_CURVE_WITH_KNOTS('',3,(#26426,#26427,#26428,#26429),
 .UNSPECIFIED.,.F.,.F.,(4,4),(-0.0821909663425472,0.),.UNSPECIFIED.);
#1179=B_SPLINE_CURVE_WITH_KNOTS('',3,(#26462,#26463,#26464,#26465),
 .UNSPECIFIED.,.F.,.F.,(4,4),(-0.0821972417992798,0.),.UNSPECIFIED.);
#1180=B_SPLINE_CURVE_WITH_KNOTS('',3,(#26473,#26474,#26475,#26476),
 .UNSPECIFIED.,.F.,.F.,(4,4),(-0.0821909663425245,0.),.UNSPECIFIED.);
#1181=B_SPLINE_CURVE_WITH_KNOTS('',3,(#26509,#26510,#26511,#26512),
 .UNSPECIFIED.,.F.,.F.,(4,4),(-0.082197241799281,0.),.UNSPECIFIED.);
#1182=B_SPLINE_CURVE_WITH_KNOTS('',3,(#26520,#26521,#26522,#26523),
 .UNSPECIFIED.,.F.,.F.,(4,4),(-0.0821909663425156,0.),.UNSPECIFIED.);
#1183=B_SPLINE_CURVE_WITH_KNOTS('',3,(#26556,#26557,#26558,#26559),
 .UNSPECIFIED.,.F.,.F.,(4,4),(-0.0821972417993007,0.),.UNSPECIFIED.);
#1184=B_SPLINE_CURVE_WITH_KNOTS('',3,(#26567,#26568,#26569,#26570),
 .UNSPECIFIED.,.F.,.F.,(4,4),(-0.082190966342518,0.),.UNSPECIFIED.);
#1185=B_SPLINE_CURVE_WITH_KNOTS('',3,(#26618,#26619,#26620,#26621),
 .UNSPECIFIED.,.F.,.F.,(4,4),(-0.0821972417993147,0.),.UNSPECIFIED.);
#1186=B_SPLINE_CURVE_WITH_KNOTS('',3,(#26629,#26630,#26631,#26632),
 .UNSPECIFIED.,.F.,.F.,(4,4),(-0.0821909663426471,0.),.UNSPECIFIED.);
#1489=CYLINDRICAL_SURFACE('',#15993,11.1);
#1490=CYLINDRICAL_SURFACE('',#16103,3.35);
#1491=CYLINDRICAL_SURFACE('',#16139,15.);
#1492=CYLINDRICAL_SURFACE('',#16143,14.);
#1493=CYLINDRICAL_SURFACE('',#16147,12.5);
#1978=FACE_OUTER_BOUND('',#2934,.T.);
#1979=FACE_OUTER_BOUND('',#2935,.T.);
#1980=FACE_OUTER_BOUND('',#2936,.T.);
#1981=FACE_OUTER_BOUND('',#2937,.T.);
#1982=FACE_OUTER_BOUND('',#2938,.T.);
#1983=FACE_OUTER_BOUND('',#2939,.T.);
#1984=FACE_OUTER_BOUND('',#2940,.T.);
#1985=FACE_OUTER_BOUND('',#2941,.T.);
#1986=FACE_OUTER_BOUND('',#2942,.T.);
#1987=FACE_OUTER_BOUND('',#2943,.T.);
#1988=FACE_OUTER_BOUND('',#2944,.T.);
#1989=FACE_OUTER_BOUND('',#2945,.T.);
#1990=FACE_OUTER_BOUND('',#2946,.T.);
#1991=FACE_OUTER_BOUND('',#2947,.T.);
#1992=FACE_OUTER_BOUND('',#2948,.T.);
#1993=FACE_OUTER_BOUND('',#2949,.T.);
#1994=FACE_OUTER_BOUND('',#2950,.T.);
#1995=FACE_OUTER_BOUND('',#2951,.T.);
#1996=FACE_OUTER_BOUND('',#2952,.T.);
#1997=FACE_OUTER_BOUND('',#2953,.T.);
#1998=FACE_OUTER_BOUND('',#2954,.T.);
#1999=FACE_OUTER_BOUND('',#2955,.T.);
#2000=FACE_OUTER_BOUND('',#2956,.T.);
#2001=FACE_OUTER_BOUND('',#2957,.T.);
#2002=FACE_OUTER_BOUND('',#2958,.T.);
#2003=FACE_OUTER_BOUND('',#2959,.T.);
#2004=FACE_OUTER_BOUND('',#2960,.T.);
#2005=FACE_OUTER_BOUND('',#2961,.T.);
#2006=FACE_OUTER_BOUND('',#2962,.T.);
#2007=FACE_OUTER_BOUND('',#2963,.T.);
#2008=FACE_OUTER_BOUND('',#2964,.T.);
#2009=FACE_OUTER_BOUND('',#2965,.T.);
#2010=FACE_OUTER_BOUND('',#2966,.T.);
#2011=FACE_OUTER_BOUND('',#2967,.T.);
#2012=FACE_OUTER_BOUND('',#2968,.T.);
#2013=FACE_OUTER_BOUND('',#2969,.T.);
#2014=FACE_OUTER_BOUND('',#2970,.T.);
#2015=FACE_OUTER_BOUND('',#2971,.T.);
#2016=FACE_OUTER_BOUND('',#2972,.T.);
#2017=FACE_OUTER_BOUND('',#2973,.T.);
#2018=FACE_OUTER_BOUND('',#2974,.T.);
#2019=FACE_OUTER_BOUND('',#2975,.T.);
#2020=FACE_OUTER_BOUND('',#2976,.T.);
#2021=FACE_OUTER_BOUND('',#2977,.T.);
#2022=FACE_OUTER_BOUND('',#2978,.T.);
#2023=FACE_OUTER_BOUND('',#2979,.T.);
#2024=FACE_OUTER_BOUND('',#2980,.T.);
#2025=FACE_OUTER_BOUND('',#2981,.T.);
#2026=FACE_OUTER_BOUND('',#2982,.T.);
#2027=FACE_OUTER_BOUND('',#2983,.T.);
#2028=FACE_OUTER_BOUND('',#2984,.T.);
#2029=FACE_OUTER_BOUND('',#2985,.T.);
#2030=FACE_OUTER_BOUND('',#2986,.T.);
#2031=FACE_OUTER_BOUND('',#2987,.T.);
#2032=FACE_OUTER_BOUND('',#2988,.T.);
#2033=FACE_OUTER_BOUND('',#2989,.T.);
#2034=FACE_OUTER_BOUND('',#2990,.T.);
#2035=FACE_OUTER_BOUND('',#2991,.T.);
#2036=FACE_OUTER_BOUND('',#2992,.T.);
#2037=FACE_OUTER_BOUND('',#2993,.T.);
#2038=FACE_OUTER_BOUND('',#2994,.T.);
#2039=FACE_OUTER_BOUND('',#2995,.T.);
#2040=FACE_OUTER_BOUND('',#2996,.T.);
#2041=FACE_OUTER_BOUND('',#2997,.T.);
#2042=FACE_OUTER_BOUND('',#2998,.T.);
#2043=FACE_OUTER_BOUND('',#2999,.T.);
#2044=FACE_OUTER_BOUND('',#3000,.T.);
#2045=FACE_OUTER_BOUND('',#3001,.T.);
#2046=FACE_OUTER_BOUND('',#3002,.T.);
#2047=FACE_OUTER_BOUND('',#3003,.T.);
#2048=FACE_OUTER_BOUND('',#3004,.T.);
#2049=FACE_OUTER_BOUND('',#3005,.T.);
#2050=FACE_OUTER_BOUND('',#3006,.T.);
#2051=FACE_OUTER_BOUND('',#3007,.T.);
#2052=FACE_OUTER_BOUND('',#3008,.T.);
#2053=FACE_OUTER_BOUND('',#3009,.T.);
#2054=FACE_OUTER_BOUND('',#3010,.T.);
#2055=FACE_OUTER_BOUND('',#3011,.T.);
#2056=FACE_OUTER_BOUND('',#3012,.T.);
#2057=FACE_OUTER_BOUND('',#3013,.T.);
#2058=FACE_OUTER_BOUND('',#3014,.T.);
#2059=FACE_OUTER_BOUND('',#3015,.T.);
#2060=FACE_OUTER_BOUND('',#3016,.T.);
#2061=FACE_OUTER_BOUND('',#3017,.T.);
#2062=FACE_OUTER_BOUND('',#3018,.T.);
#2063=FACE_OUTER_BOUND('',#3019,.T.);
#2064=FACE_OUTER_BOUND('',#3020,.T.);
#2065=FACE_OUTER_BOUND('',#3021,.T.);
#2066=FACE_OUTER_BOUND('',#3022,.T.);
#2067=FACE_OUTER_BOUND('',#3023,.T.);
#2068=FACE_OUTER_BOUND('',#3024,.T.);
#2069=FACE_OUTER_BOUND('',#3025,.T.);
#2070=FACE_OUTER_BOUND('',#3026,.T.);
#2071=FACE_OUTER_BOUND('',#3027,.T.);
#2072=FACE_OUTER_BOUND('',#3028,.T.);
#2073=FACE_OUTER_BOUND('',#3029,.T.);
#2074=FACE_OUTER_BOUND('',#3030,.T.);
#2075=FACE_OUTER_BOUND('',#3031,.T.);
#2076=FACE_OUTER_BOUND('',#3032,.T.);
#2077=FACE_OUTER_BOUND('',#3033,.T.);
#2078=FACE_OUTER_BOUND('',#3034,.T.);
#2079=FACE_OUTER_BOUND('',#3035,.T.);
#2080=FACE_OUTER_BOUND('',#3036,.T.);
#2081=FACE_OUTER_BOUND('',#3037,.T.);
#2082=FACE_OUTER_BOUND('',#3038,.T.);
#2083=FACE_OUTER_BOUND('',#3039,.T.);
#2084=FACE_OUTER_BOUND('',#3040,.T.);
#2085=FACE_OUTER_BOUND('',#3041,.T.);
#2086=FACE_OUTER_BOUND('',#3043,.T.);
#2087=FACE_OUTER_BOUND('',#3044,.T.);
#2088=FACE_OUTER_BOUND('',#3045,.T.);
#2089=FACE_OUTER_BOUND('',#3046,.T.);
#2090=FACE_OUTER_BOUND('',#3047,.T.);
#2091=FACE_OUTER_BOUND('',#3048,.T.);
#2092=FACE_OUTER_BOUND('',#3049,.T.);
#2093=FACE_OUTER_BOUND('',#3050,.T.);
#2094=FACE_OUTER_BOUND('',#3051,.T.);
#2095=FACE_OUTER_BOUND('',#3052,.T.);
#2096=FACE_OUTER_BOUND('',#3053,.T.);
#2097=FACE_OUTER_BOUND('',#3054,.T.);
#2098=FACE_OUTER_BOUND('',#3055,.T.);
#2099=FACE_OUTER_BOUND('',#3056,.T.);
#2100=FACE_OUTER_BOUND('',#3057,.T.);
#2101=FACE_OUTER_BOUND('',#3058,.T.);
#2102=FACE_OUTER_BOUND('',#3059,.T.);
#2103=FACE_OUTER_BOUND('',#3060,.T.);
#2104=FACE_OUTER_BOUND('',#3061,.T.);
#2105=FACE_OUTER_BOUND('',#3062,.T.);
#2106=FACE_OUTER_BOUND('',#3064,.T.);
#2107=FACE_OUTER_BOUND('',#3065,.T.);
#2108=FACE_OUTER_BOUND('',#3067,.T.);
#2109=FACE_OUTER_BOUND('',#3068,.T.);
#2110=FACE_OUTER_BOUND('',#3070,.T.);
#2111=FACE_OUTER_BOUND('',#3072,.T.);
#2112=FACE_OUTER_BOUND('',#3073,.T.);
#2934=EDGE_LOOP('',(#11497,#11498,#11499,#11500));
#2935=EDGE_LOOP('',(#11501,#11502,#11503,#11504));
#2936=EDGE_LOOP('',(#11505,#11506,#11507,#11508,#11509,#11510));
#2937=EDGE_LOOP('',(#11511,#11512,#11513,#11514,#11515,#11516,#11517));
#2938=EDGE_LOOP('',(#11518,#11519,#11520,#11521));
#2939=EDGE_LOOP('',(#11522,#11523,#11524,#11525,#11526,#11527,#11528));
#2940=EDGE_LOOP('',(#11529,#11530,#11531,#11532));
#2941=EDGE_LOOP('',(#11533,#11534,#11535,#11536));
#2942=EDGE_LOOP('',(#11537,#11538,#11539,#11540,#11541,#11542));
#2943=EDGE_LOOP('',(#11543,#11544,#11545,#11546,#11547,#11548,#11549));
#2944=EDGE_LOOP('',(#11550,#11551,#11552,#11553));
#2945=EDGE_LOOP('',(#11554,#11555,#11556,#11557,#11558,#11559,#11560));
#2946=EDGE_LOOP('',(#11561,#11562,#11563,#11564));
#2947=EDGE_LOOP('',(#11565,#11566,#11567,#11568));
#2948=EDGE_LOOP('',(#11569,#11570,#11571,#11572,#11573,#11574));
#2949=EDGE_LOOP('',(#11575,#11576,#11577,#11578,#11579,#11580,#11581));
#2950=EDGE_LOOP('',(#11582,#11583,#11584,#11585));
#2951=EDGE_LOOP('',(#11586,#11587,#11588,#11589,#11590,#11591,#11592));
#2952=EDGE_LOOP('',(#11593,#11594,#11595,#11596));
#2953=EDGE_LOOP('',(#11597,#11598,#11599,#11600));
#2954=EDGE_LOOP('',(#11601,#11602,#11603,#11604,#11605,#11606));
#2955=EDGE_LOOP('',(#11607,#11608,#11609,#11610,#11611,#11612,#11613));
#2956=EDGE_LOOP('',(#11614,#11615,#11616,#11617));
#2957=EDGE_LOOP('',(#11618,#11619,#11620,#11621,#11622,#11623,#11624));
#2958=EDGE_LOOP('',(#11625,#11626,#11627,#11628));
#2959=EDGE_LOOP('',(#11629,#11630,#11631,#11632,#11633,#11634,#11635));
#2960=EDGE_LOOP('',(#11636,#11637,#11638,#11639));
#2961=EDGE_LOOP('',(#11640,#11641,#11642,#11643,#11644,#11645));
#2962=EDGE_LOOP('',(#11646,#11647,#11648,#11649,#11650,#11651,#11652));
#2963=EDGE_LOOP('',(#11653,#11654,#11655,#11656,#11657,#11658));
#2964=EDGE_LOOP('',(#11659,#11660,#11661,#11662,#11663,#11664,#11665,#11666,
#11667,#11668,#11669,#11670,#11671,#11672,#11673,#11674,#11675,#11676,#11677,
#11678,#11679,#11680,#11681,#11682,#11683,#11684,#11685,#11686,#11687,#11688,
#11689,#11690,#11691,#11692,#11693,#11694,#11695,#11696,#11697,#11698,#11699,
#11700,#11701,#11702,#11703,#11704,#11705,#11706,#11707,#11708,#11709,#11710,
#11711,#11712,#11713,#11714));
#2965=EDGE_LOOP('',(#11715,#11716,#11717,#11718));
#2966=EDGE_LOOP('',(#11719,#11720,#11721,#11722));
#2967=EDGE_LOOP('',(#11723,#11724,#11725,#11726,#11727,#11728));
#2968=EDGE_LOOP('',(#11729,#11730,#11731,#11732,#11733,#11734,#11735));
#2969=EDGE_LOOP('',(#11736,#11737,#11738,#11739));
#2970=EDGE_LOOP('',(#11740,#11741,#11742,#11743,#11744,#11745,#11746));
#2971=EDGE_LOOP('',(#11747,#11748,#11749,#11750));
#2972=EDGE_LOOP('',(#11751,#11752,#11753,#11754));
#2973=EDGE_LOOP('',(#11755,#11756,#11757,#11758,#11759,#11760));
#2974=EDGE_LOOP('',(#11761,#11762,#11763,#11764,#11765,#11766,#11767));
#2975=EDGE_LOOP('',(#11768,#11769,#11770,#11771));
#2976=EDGE_LOOP('',(#11772,#11773,#11774,#11775,#11776,#11777,#11778));
#2977=EDGE_LOOP('',(#11779,#11780,#11781,#11782));
#2978=EDGE_LOOP('',(#11783,#11784,#11785,#11786));
#2979=EDGE_LOOP('',(#11787,#11788,#11789,#11790));
#2980=EDGE_LOOP('',(#11791,#11792,#11793,#11794));
#2981=EDGE_LOOP('',(#11795,#11796,#11797,#11798));
#2982=EDGE_LOOP('',(#11799,#11800,#11801,#11802));
#2983=EDGE_LOOP('',(#11803,#11804,#11805,#11806));
#2984=EDGE_LOOP('',(#11807,#11808,#11809,#11810));
#2985=EDGE_LOOP('',(#11811,#11812,#11813,#11814));
#2986=EDGE_LOOP('',(#11815,#11816,#11817,#11818));
#2987=EDGE_LOOP('',(#11819,#11820,#11821,#11822));
#2988=EDGE_LOOP('',(#11823,#11824,#11825,#11826));
#2989=EDGE_LOOP('',(#11827,#11828,#11829,#11830));
#2990=EDGE_LOOP('',(#11831,#11832,#11833,#11834));
#2991=EDGE_LOOP('',(#11835,#11836,#11837,#11838));
#2992=EDGE_LOOP('',(#11839,#11840,#11841,#11842));
#2993=EDGE_LOOP('',(#11843,#11844,#11845,#11846));
#2994=EDGE_LOOP('',(#11847,#11848,#11849,#11850));
#2995=EDGE_LOOP('',(#11851,#11852,#11853,#11854));
#2996=EDGE_LOOP('',(#11855,#11856,#11857,#11858));
#2997=EDGE_LOOP('',(#11859,#11860,#11861,#11862));
#2998=EDGE_LOOP('',(#11863,#11864,#11865,#11866));
#2999=EDGE_LOOP('',(#11867,#11868,#11869,#11870));
#3000=EDGE_LOOP('',(#11871,#11872,#11873,#11874));
#3001=EDGE_LOOP('',(#11875,#11876,#11877,#11878));
#3002=EDGE_LOOP('',(#11879,#11880,#11881,#11882));
#3003=EDGE_LOOP('',(#11883,#11884,#11885,#11886,#11887,#11888));
#3004=EDGE_LOOP('',(#11889,#11890,#11891,#11892,#11893,#11894,#11895));
#3005=EDGE_LOOP('',(#11896,#11897,#11898,#11899));
#3006=EDGE_LOOP('',(#11900,#11901,#11902,#11903,#11904,#11905,#11906));
#3007=EDGE_LOOP('',(#11907,#11908,#11909,#11910));
#3008=EDGE_LOOP('',(#11911,#11912,#11913,#11914));
#3009=EDGE_LOOP('',(#11915,#11916,#11917,#11918,#11919,#11920,#11921));
#3010=EDGE_LOOP('',(#11922,#11923,#11924,#11925,#11926,#11927,#11928));
#3011=EDGE_LOOP('',(#11929,#11930,#11931,#11932));
#3012=EDGE_LOOP('',(#11933,#11934,#11935,#11936,#11937,#11938,#11939));
#3013=EDGE_LOOP('',(#11940,#11941,#11942,#11943));
#3014=EDGE_LOOP('',(#11944,#11945,#11946,#11947));
#3015=EDGE_LOOP('',(#11948,#11949,#11950,#11951,#11952,#11953));
#3016=EDGE_LOOP('',(#11954,#11955,#11956,#11957,#11958,#11959,#11960));
#3017=EDGE_LOOP('',(#11961,#11962,#11963,#11964));
#3018=EDGE_LOOP('',(#11965,#11966,#11967,#11968,#11969,#11970,#11971));
#3019=EDGE_LOOP('',(#11972,#11973,#11974,#11975));
#3020=EDGE_LOOP('',(#11976,#11977,#11978,#11979));
#3021=EDGE_LOOP('',(#11980,#11981,#11982,#11983,#11984,#11985));
#3022=EDGE_LOOP('',(#11986,#11987,#11988,#11989,#11990,#11991,#11992));
#3023=EDGE_LOOP('',(#11993,#11994,#11995,#11996));
#3024=EDGE_LOOP('',(#11997,#11998,#11999,#12000,#12001,#12002,#12003));
#3025=EDGE_LOOP('',(#12004,#12005,#12006,#12007));
#3026=EDGE_LOOP('',(#12008,#12009,#12010,#12011));
#3027=EDGE_LOOP('',(#12012,#12013,#12014,#12015,#12016,#12017));
#3028=EDGE_LOOP('',(#12018,#12019,#12020,#12021));
#3029=EDGE_LOOP('',(#12022,#12023,#12024,#12025,#12026,#12027,#12028));
#3030=EDGE_LOOP('',(#12029,#12030,#12031,#12032,#12033,#12034));
#3031=EDGE_LOOP('',(#12035,#12036,#12037,#12038));
#3032=EDGE_LOOP('',(#12039,#12040,#12041,#12042));
#3033=EDGE_LOOP('',(#12043,#12044,#12045,#12046));
#3034=EDGE_LOOP('',(#12047,#12048,#12049,#12050));
#3035=EDGE_LOOP('',(#12051,#12052,#12053,#12054,#12055,#12056));
#3036=EDGE_LOOP('',(#12057,#12058,#12059,#12060));
#3037=EDGE_LOOP('',(#12061,#12062,#12063,#12064,#12065,#12066,#12067));
#3038=EDGE_LOOP('',(#12068,#12069,#12070,#12071,#12072,#12073));
#3039=EDGE_LOOP('',(#12074,#12075,#12076,#12077));
#3040=EDGE_LOOP('',(#12078,#12079,#12080,#12081));
#3041=EDGE_LOOP('',(#12082,#12083,#12084,#12085,#12086,#12087,#12088,#12089,
#12090,#12091,#12092,#12093,#12094,#12095,#12096,#12097,#12098,#12099,#12100,
#12101,#12102,#12103,#12104,#12105,#12106,#12107,#12108,#12109,#12110,#12111,
#12112,#12113,#12114,#12115,#12116,#12117,#12118,#12119,#12120,#12121,#12122,
#12123,#12124,#12125,#12126,#12127,#12128,#12129,#12130,#12131,#12132,#12133));
#3042=EDGE_LOOP('',(#12134));
#3043=EDGE_LOOP('',(#12135));
#3044=EDGE_LOOP('',(#12136,#12137,#12138,#12139));
#3045=EDGE_LOOP('',(#12140,#12141,#12142,#12143));
#3046=EDGE_LOOP('',(#12144,#12145,#12146,#12147));
#3047=EDGE_LOOP('',(#12148,#12149,#12150,#12151));
#3048=EDGE_LOOP('',(#12152,#12153,#12154,#12155));
#3049=EDGE_LOOP('',(#12156,#12157,#12158,#12159,#12160,#12161,#12162));
#3050=EDGE_LOOP('',(#12163,#12164,#12165,#12166,#12167,#12168));
#3051=EDGE_LOOP('',(#12169,#12170,#12171,#12172,#12173,#12174));
#3052=EDGE_LOOP('',(#12175,#12176,#12177,#12178,#12179,#12180));
#3053=EDGE_LOOP('',(#12181,#12182,#12183,#12184,#12185,#12186));
#3054=EDGE_LOOP('',(#12187,#12188,#12189,#12190));
#3055=EDGE_LOOP('',(#12191,#12192,#12193,#12194,#12195,#12196));
#3056=EDGE_LOOP('',(#12197,#12198,#12199,#12200,#12201,#12202));
#3057=EDGE_LOOP('',(#12203,#12204,#12205,#12206,#12207,#12208));
#3058=EDGE_LOOP('',(#12209,#12210,#12211,#12212,#12213,#12214));
#3059=EDGE_LOOP('',(#12215,#12216,#12217,#12218,#12219,#12220));
#3060=EDGE_LOOP('',(#12221,#12222,#12223,#12224,#12225,#12226,#12227));
#3061=EDGE_LOOP('',(#12228,#12229,#12230,#12231,#12232,#12233));
#3062=EDGE_LOOP('',(#12234));
#3063=EDGE_LOOP('',(#12235));
#3064=EDGE_LOOP('',(#12236,#12237,#12238,#12239));
#3065=EDGE_LOOP('',(#12240));
#3066=EDGE_LOOP('',(#12241));
#3067=EDGE_LOOP('',(#12242,#12243,#12244,#12245));
#3068=EDGE_LOOP('',(#12246));
#3069=EDGE_LOOP('',(#12247));
#3070=EDGE_LOOP('',(#12248,#12249,#12250,#12251));
#3071=EDGE_LOOP('',(#12252,#12253,#12254,#12255));
#3072=EDGE_LOOP('',(#12256,#12257,#12258,#12259));
#3073=EDGE_LOOP('',(#12260));
#3846=LINE('',#25745,#4915);
#3847=LINE('',#25751,#4916);
#3848=LINE('',#25759,#4917);
#3849=LINE('',#25765,#4918);
#3850=LINE('',#25783,#4919);
#3851=LINE('',#25785,#4920);
#3852=LINE('',#25787,#4921);
#3853=LINE('',#25789,#4922);
#3854=LINE('',#25795,#4923);
#3855=LINE('',#25796,#4924);
#3856=LINE('',#25803,#4925);
#3857=LINE('',#25805,#4926);
#3858=LINE('',#25806,#4927);
#3859=LINE('',#25810,#4928);
#3860=LINE('',#25816,#4929);
#3861=LINE('',#25824,#4930);
#3862=LINE('',#25830,#4931);
#3863=LINE('',#25848,#4932);
#3864=LINE('',#25850,#4933);
#3865=LINE('',#25852,#4934);
#3866=LINE('',#25854,#4935);
#3867=LINE('',#25860,#4936);
#3868=LINE('',#25861,#4937);
#3869=LINE('',#25868,#4938);
#3870=LINE('',#25870,#4939);
#3871=LINE('',#25871,#4940);
#3872=LINE('',#25875,#4941);
#3873=LINE('',#25881,#4942);
#3874=LINE('',#25889,#4943);
#3875=LINE('',#25895,#4944);
#3876=LINE('',#25913,#4945);
#3877=LINE('',#25915,#4946);
#3878=LINE('',#25917,#4947);
#3879=LINE('',#25919,#4948);
#3880=LINE('',#25925,#4949);
#3881=LINE('',#25926,#4950);
#3882=LINE('',#25933,#4951);
#3883=LINE('',#25935,#4952);
#3884=LINE('',#25936,#4953);
#3885=LINE('',#25940,#4954);
#3886=LINE('',#25946,#4955);
#3887=LINE('',#25954,#4956);
#3888=LINE('',#25960,#4957);
#3889=LINE('',#25978,#4958);
#3890=LINE('',#25980,#4959);
#3891=LINE('',#25982,#4960);
#3892=LINE('',#25984,#4961);
#3893=LINE('',#25990,#4962);
#3894=LINE('',#25991,#4963);
#3895=LINE('',#25998,#4964);
#3896=LINE('',#26000,#4965);
#3897=LINE('',#26001,#4966);
#3898=LINE('',#26009,#4967);
#3899=LINE('',#26014,#4968);
#3900=LINE('',#26021,#4969);
#3901=LINE('',#26023,#4970);
#3902=LINE('',#26025,#4971);
#3903=LINE('',#26027,#4972);
#3904=LINE('',#26034,#4973);
#3905=LINE('',#26040,#4974);
#3906=LINE('',#26058,#4975);
#3907=LINE('',#26060,#4976);
#3908=LINE('',#26062,#4977);
#3909=LINE('',#26063,#4978);
#3910=LINE('',#26080,#4979);
#3911=LINE('',#26084,#4980);
#3912=LINE('',#26088,#4981);
#3913=LINE('',#26092,#4982);
#3914=LINE('',#26096,#4983);
#3915=LINE('',#26100,#4984);
#3916=LINE('',#26104,#4985);
#3917=LINE('',#26107,#4986);
#3918=LINE('',#26115,#4987);
#3919=LINE('',#26119,#4988);
#3920=LINE('',#26123,#4989);
#3921=LINE('',#26127,#4990);
#3922=LINE('',#26131,#4991);
#3923=LINE('',#26135,#4992);
#3924=LINE('',#26139,#4993);
#3925=LINE('',#26143,#4994);
#3926=LINE('',#26147,#4995);
#3927=LINE('',#26151,#4996);
#3928=LINE('',#26162,#4997);
#3929=LINE('',#26179,#4998);
#3930=LINE('',#26181,#4999);
#3931=LINE('',#26183,#5000);
#3932=LINE('',#26184,#5001);
#3933=LINE('',#26187,#5002);
#3934=LINE('',#26188,#5003);
#3935=LINE('',#26195,#5004);
#3936=LINE('',#26197,#5005);
#3937=LINE('',#26198,#5006);
#3938=LINE('',#26202,#5007);
#3939=LINE('',#26216,#5008);
#3940=LINE('',#26233,#5009);
#3941=LINE('',#26235,#5010);
#3942=LINE('',#26237,#5011);
#3943=LINE('',#26239,#5012);
#3944=LINE('',#26245,#5013);
#3945=LINE('',#26246,#5014);
#3946=LINE('',#26253,#5015);
#3947=LINE('',#26255,#5016);
#3948=LINE('',#26256,#5017);
#3949=LINE('',#26260,#5018);
#3950=LINE('',#26262,#5019);
#3951=LINE('',#26264,#5020);
#3952=LINE('',#26265,#5021);
#3953=LINE('',#26268,#5022);
#3954=LINE('',#26270,#5023);
#3955=LINE('',#26271,#5024);
#3956=LINE('',#26275,#5025);
#3957=LINE('',#26277,#5026);
#3958=LINE('',#26279,#5027);
#3959=LINE('',#26280,#5028);
#3960=LINE('',#26283,#5029);
#3961=LINE('',#26285,#5030);
#3962=LINE('',#26286,#5031);
#3963=LINE('',#26290,#5032);
#3964=LINE('',#26292,#5033);
#3965=LINE('',#26294,#5034);
#3966=LINE('',#26295,#5035);
#3967=LINE('',#26298,#5036);
#3968=LINE('',#26300,#5037);
#3969=LINE('',#26301,#5038);
#3970=LINE('',#26305,#5039);
#3971=LINE('',#26307,#5040);
#3972=LINE('',#26309,#5041);
#3973=LINE('',#26310,#5042);
#3974=LINE('',#26313,#5043);
#3975=LINE('',#26315,#5044);
#3976=LINE('',#26316,#5045);
#3977=LINE('',#26320,#5046);
#3978=LINE('',#26322,#5047);
#3979=LINE('',#26324,#5048);
#3980=LINE('',#26325,#5049);
#3981=LINE('',#26328,#5050);
#3982=LINE('',#26330,#5051);
#3983=LINE('',#26331,#5052);
#3984=LINE('',#26333,#5053);
#3985=LINE('',#26334,#5054);
#3986=LINE('',#26337,#5055);
#3987=LINE('',#26338,#5056);
#3988=LINE('',#26341,#5057);
#3989=LINE('',#26342,#5058);
#3990=LINE('',#26344,#5059);
#3991=LINE('',#26346,#5060);
#3992=LINE('',#26347,#5061);
#3993=LINE('',#26350,#5062);
#3994=LINE('',#26351,#5063);
#3995=LINE('',#26354,#5064);
#3996=LINE('',#26355,#5065);
#3997=LINE('',#26358,#5066);
#3998=LINE('',#26359,#5067);
#3999=LINE('',#26364,#5068);
#4000=LINE('',#26378,#5069);
#4001=LINE('',#26394,#5070);
#4002=LINE('',#26396,#5071);
#4003=LINE('',#26401,#5072);
#4004=LINE('',#26407,#5073);
#4005=LINE('',#26411,#5074);
#4006=LINE('',#26425,#5075);
#4007=LINE('',#26441,#5076);
#4008=LINE('',#26443,#5077);
#4009=LINE('',#26448,#5078);
#4010=LINE('',#26454,#5079);
#4011=LINE('',#26458,#5080);
#4012=LINE('',#26472,#5081);
#4013=LINE('',#26488,#5082);
#4014=LINE('',#26490,#5083);
#4015=LINE('',#26495,#5084);
#4016=LINE('',#26501,#5085);
#4017=LINE('',#26505,#5086);
#4018=LINE('',#26519,#5087);
#4019=LINE('',#26535,#5088);
#4020=LINE('',#26537,#5089);
#4021=LINE('',#26542,#5090);
#4022=LINE('',#26548,#5091);
#4023=LINE('',#26552,#5092);
#4024=LINE('',#26566,#5093);
#4025=LINE('',#26582,#5094);
#4026=LINE('',#26583,#5095);
#4027=LINE('',#26589,#5096);
#4028=LINE('',#26603,#5097);
#4029=LINE('',#26605,#5098);
#4030=LINE('',#26607,#5099);
#4031=LINE('',#26608,#5100);
#4032=LINE('',#26611,#5101);
#4033=LINE('',#26613,#5102);
#4034=LINE('',#26614,#5103);
#4035=LINE('',#26617,#5104);
#4036=LINE('',#26628,#5105);
#4037=LINE('',#26644,#5106);
#4038=LINE('',#26645,#5107);
#4039=LINE('',#26651,#5108);
#4040=LINE('',#26658,#5109);
#4041=LINE('',#26662,#5110);
#4042=LINE('',#26665,#5111);
#4043=LINE('',#26677,#5112);
#4044=LINE('',#26684,#5113);
#4045=LINE('',#26686,#5114);
#4046=LINE('',#26687,#5115);
#4047=LINE('',#26690,#5116);
#4048=LINE('',#26692,#5117);
#4049=LINE('',#26693,#5118);
#4050=LINE('',#26696,#5119);
#4051=LINE('',#26698,#5120);
#4052=LINE('',#26699,#5121);
#4053=LINE('',#26702,#5122);
#4054=LINE('',#26726,#5123);
#4055=LINE('',#26733,#5124);
#4056=LINE('',#26740,#5125);
#4057=LINE('',#26744,#5126);
#4915=VECTOR('',#18489,10.);
#4916=VECTOR('',#18490,10.);
#4917=VECTOR('',#18493,10.);
#4918=VECTOR('',#18494,10.);
#4919=VECTOR('',#18503,10.);
#4920=VECTOR('',#18504,10.);
#4921=VECTOR('',#18505,10.);
#4922=VECTOR('',#18506,10.);
#4923=VECTOR('',#18509,10.);
#4924=VECTOR('',#18510,10.);
#4925=VECTOR('',#18513,10.);
#4926=VECTOR('',#18514,10.);
#4927=VECTOR('',#18515,10.);
#4928=VECTOR('',#18518,10.);
#4929=VECTOR('',#18519,10.);
#4930=VECTOR('',#18522,10.);
#4931=VECTOR('',#18523,10.);
#4932=VECTOR('',#18532,10.);
#4933=VECTOR('',#18533,10.);
#4934=VECTOR('',#18534,10.);
#4935=VECTOR('',#18535,10.);
#4936=VECTOR('',#18538,10.);
#4937=VECTOR('',#18539,10.);
#4938=VECTOR('',#18542,10.);
#4939=VECTOR('',#18543,10.);
#4940=VECTOR('',#18544,10.);
#4941=VECTOR('',#18547,10.);
#4942=VECTOR('',#18548,10.);
#4943=VECTOR('',#18551,10.);
#4944=VECTOR('',#18552,10.);
#4945=VECTOR('',#18561,10.);
#4946=VECTOR('',#18562,10.);
#4947=VECTOR('',#18563,10.);
#4948=VECTOR('',#18564,10.);
#4949=VECTOR('',#18567,10.);
#4950=VECTOR('',#18568,10.);
#4951=VECTOR('',#18571,10.);
#4952=VECTOR('',#18572,10.);
#4953=VECTOR('',#18573,10.);
#4954=VECTOR('',#18576,10.);
#4955=VECTOR('',#18577,10.);
#4956=VECTOR('',#18580,10.);
#4957=VECTOR('',#18581,10.);
#4958=VECTOR('',#18590,10.);
#4959=VECTOR('',#18591,10.);
#4960=VECTOR('',#18592,10.);
#4961=VECTOR('',#18593,10.);
#4962=VECTOR('',#18596,10.);
#4963=VECTOR('',#18597,10.);
#4964=VECTOR('',#18600,10.);
#4965=VECTOR('',#18601,10.);
#4966=VECTOR('',#18602,10.);
#4967=VECTOR('',#18605,10.);
#4968=VECTOR('',#18606,10.);
#4969=VECTOR('',#18609,10.);
#4970=VECTOR('',#18610,10.);
#4971=VECTOR('',#18611,10.);
#4972=VECTOR('',#18612,10.);
#4973=VECTOR('',#18615,10.);
#4974=VECTOR('',#18616,10.);
#4975=VECTOR('',#18625,10.);
#4976=VECTOR('',#18626,10.);
#4977=VECTOR('',#18627,10.);
#4978=VECTOR('',#18628,10.);
#4979=VECTOR('',#18639,11.1);
#4980=VECTOR('',#18642,10.);
#4981=VECTOR('',#18645,10.);
#4982=VECTOR('',#18648,10.);
#4983=VECTOR('',#18651,10.);
#4984=VECTOR('',#18654,10.);
#4985=VECTOR('',#18657,10.);
#4986=VECTOR('',#18660,10.);
#4987=VECTOR('',#18671,10.);
#4988=VECTOR('',#18674,10.);
#4989=VECTOR('',#18677,10.);
#4990=VECTOR('',#18680,10.);
#4991=VECTOR('',#18683,10.);
#4992=VECTOR('',#18686,10.);
#4993=VECTOR('',#18689,10.);
#4994=VECTOR('',#18692,10.);
#4995=VECTOR('',#18695,10.);
#4996=VECTOR('',#18700,10.);
#4997=VECTOR('',#18703,10.);
#4998=VECTOR('',#18710,10.);
#4999=VECTOR('',#18711,10.);
#5000=VECTOR('',#18712,10.);
#5001=VECTOR('',#18713,10.);
#5002=VECTOR('',#18716,10.);
#5003=VECTOR('',#18717,10.);
#5004=VECTOR('',#18720,10.);
#5005=VECTOR('',#18721,10.);
#5006=VECTOR('',#18722,10.);
#5007=VECTOR('',#18725,10.);
#5008=VECTOR('',#18728,10.);
#5009=VECTOR('',#18735,10.);
#5010=VECTOR('',#18736,10.);
#5011=VECTOR('',#18737,10.);
#5012=VECTOR('',#18738,10.);
#5013=VECTOR('',#18741,10.);
#5014=VECTOR('',#18742,10.);
#5015=VECTOR('',#18745,10.);
#5016=VECTOR('',#18746,10.);
#5017=VECTOR('',#18747,10.);
#5018=VECTOR('',#18750,10.);
#5019=VECTOR('',#18751,10.);
#5020=VECTOR('',#18752,10.);
#5021=VECTOR('',#18753,10.);
#5022=VECTOR('',#18756,10.);
#5023=VECTOR('',#18757,10.);
#5024=VECTOR('',#18758,10.);
#5025=VECTOR('',#18761,10.);
#5026=VECTOR('',#18762,10.);
#5027=VECTOR('',#18763,10.);
#5028=VECTOR('',#18764,10.);
#5029=VECTOR('',#18767,10.);
#5030=VECTOR('',#18768,10.);
#5031=VECTOR('',#18769,10.);
#5032=VECTOR('',#18772,10.);
#5033=VECTOR('',#18773,10.);
#5034=VECTOR('',#18774,10.);
#5035=VECTOR('',#18775,10.);
#5036=VECTOR('',#18778,10.);
#5037=VECTOR('',#18779,10.);
#5038=VECTOR('',#18780,10.);
#5039=VECTOR('',#18783,10.);
#5040=VECTOR('',#18784,10.);
#5041=VECTOR('',#18785,10.);
#5042=VECTOR('',#18786,10.);
#5043=VECTOR('',#18789,10.);
#5044=VECTOR('',#18790,10.);
#5045=VECTOR('',#18791,10.);
#5046=VECTOR('',#18794,10.);
#5047=VECTOR('',#18795,10.);
#5048=VECTOR('',#18796,10.);
#5049=VECTOR('',#18797,10.);
#5050=VECTOR('',#18800,10.);
#5051=VECTOR('',#18801,10.);
#5052=VECTOR('',#18802,10.);
#5053=VECTOR('',#18805,10.);
#5054=VECTOR('',#18806,10.);
#5055=VECTOR('',#18811,10.);
#5056=VECTOR('',#18812,10.);
#5057=VECTOR('',#18817,10.);
#5058=VECTOR('',#18818,10.);
#5059=VECTOR('',#18821,10.);
#5060=VECTOR('',#18824,10.);
#5061=VECTOR('',#18825,10.);
#5062=VECTOR('',#18830,10.);
#5063=VECTOR('',#18831,10.);
#5064=VECTOR('',#18836,10.);
#5065=VECTOR('',#18837,10.);
#5066=VECTOR('',#18842,10.);
#5067=VECTOR('',#18843,10.);
#5068=VECTOR('',#18848,10.);
#5069=VECTOR('',#18851,10.);
#5070=VECTOR('',#18858,10.);
#5071=VECTOR('',#18859,10.);
#5072=VECTOR('',#18862,10.);
#5073=VECTOR('',#18865,10.);
#5074=VECTOR('',#18868,10.);
#5075=VECTOR('',#18871,10.);
#5076=VECTOR('',#18878,10.);
#5077=VECTOR('',#18879,10.);
#5078=VECTOR('',#18882,10.);
#5079=VECTOR('',#18885,10.);
#5080=VECTOR('',#18888,10.);
#5081=VECTOR('',#18891,10.);
#5082=VECTOR('',#18898,10.);
#5083=VECTOR('',#18899,10.);
#5084=VECTOR('',#18902,10.);
#5085=VECTOR('',#18905,10.);
#5086=VECTOR('',#18908,10.);
#5087=VECTOR('',#18911,10.);
#5088=VECTOR('',#18918,10.);
#5089=VECTOR('',#18919,10.);
#5090=VECTOR('',#18922,10.);
#5091=VECTOR('',#18925,10.);
#5092=VECTOR('',#18928,10.);
#5093=VECTOR('',#18931,10.);
#5094=VECTOR('',#18938,10.);
#5095=VECTOR('',#18939,10.);
#5096=VECTOR('',#18942,10.);
#5097=VECTOR('',#18949,10.);
#5098=VECTOR('',#18950,10.);
#5099=VECTOR('',#18951,10.);
#5100=VECTOR('',#18952,10.);
#5101=VECTOR('',#18955,10.);
#5102=VECTOR('',#18956,10.);
#5103=VECTOR('',#18957,10.);
#5104=VECTOR('',#18960,10.);
#5105=VECTOR('',#18963,10.);
#5106=VECTOR('',#18970,10.);
#5107=VECTOR('',#18971,10.);
#5108=VECTOR('',#18974,10.);
#5109=VECTOR('',#18983,3.6);
#5110=VECTOR('',#18988,3.35);
#5111=VECTOR('',#18993,10.);
#5112=VECTOR('',#19014,10.);
#5113=VECTOR('',#19021,10.);
#5114=VECTOR('',#19022,10.);
#5115=VECTOR('',#19023,10.);
#5116=VECTOR('',#19026,10.);
#5117=VECTOR('',#19027,10.);
#5118=VECTOR('',#19028,10.);
#5119=VECTOR('',#19031,10.);
#5120=VECTOR('',#19032,10.);
#5121=VECTOR('',#19033,10.);
#5122=VECTOR('',#19038,10.);
#5123=VECTOR('',#19075,15.);
#5124=VECTOR('',#19084,14.);
#5125=VECTOR('',#19093,12.5);
#5126=VECTOR('',#19098,12.25);
#6007=CIRCLE('',#15954,11.1);
#6008=CIRCLE('',#15955,10.6);
#6009=CIRCLE('',#15962,11.1);
#6010=CIRCLE('',#15963,10.6);
#6011=CIRCLE('',#15970,11.1);
#6012=CIRCLE('',#15971,10.6);
#6013=CIRCLE('',#15978,11.1);
#6014=CIRCLE('',#15979,10.6);
#6015=CIRCLE('',#15987,10.6);
#6016=CIRCLE('',#15988,11.1);
#6017=CIRCLE('',#15991,11.1);
#6018=CIRCLE('',#15992,10.6);
#6019=CIRCLE('',#15994,11.1);
#6020=CIRCLE('',#15995,11.1);
#6021=CIRCLE('',#15996,11.1);
#6022=CIRCLE('',#15997,11.1);
#6023=CIRCLE('',#15998,11.1);
#6024=CIRCLE('',#15999,11.1);
#6025=CIRCLE('',#16000,11.1);
#6026=CIRCLE('',#16001,11.1);
#6027=CIRCLE('',#16002,11.1);
#6028=CIRCLE('',#16003,11.1);
#6029=CIRCLE('',#16004,11.1);
#6030=CIRCLE('',#16005,11.1);
#6031=CIRCLE('',#16006,11.1);
#6032=CIRCLE('',#16007,11.1);
#6033=CIRCLE('',#16008,11.1);
#6034=CIRCLE('',#16009,11.1);
#6035=CIRCLE('',#16010,11.1);
#6036=CIRCLE('',#16011,11.1);
#6037=CIRCLE('',#16012,11.1);
#6038=CIRCLE('',#16013,11.1);
#6039=CIRCLE('',#16014,11.1);
#6040=CIRCLE('',#16015,11.1);
#6041=CIRCLE('',#16019,10.6);
#6042=CIRCLE('',#16026,10.6);
#6043=CIRCLE('',#16057,10.6);
#6044=CIRCLE('',#16064,10.6);
#6045=CIRCLE('',#16071,10.6);
#6046=CIRCLE('',#16078,10.6);
#6047=CIRCLE('',#16085,10.6);
#6048=CIRCLE('',#16089,10.6);
#6049=CIRCLE('',#16095,10.6);
#6050=CIRCLE('',#16099,10.6);
#6051=CIRCLE('',#16101,3.85);
#6052=CIRCLE('',#16102,3.35);
#6053=CIRCLE('',#16104,3.35);
#6054=CIRCLE('',#16106,10.6);
#6055=CIRCLE('',#16107,10.6);
#6056=CIRCLE('',#16108,10.6);
#6057=CIRCLE('',#16109,10.6);
#6058=CIRCLE('',#16110,10.6);
#6059=CIRCLE('',#16111,10.6);
#6060=CIRCLE('',#16112,10.6);
#6061=CIRCLE('',#16113,10.6);
#6062=CIRCLE('',#16114,10.6);
#6063=CIRCLE('',#16115,10.6);
#6064=CIRCLE('',#16118,12.5);
#6065=CIRCLE('',#16122,12.5);
#6066=CIRCLE('',#16138,15.);
#6067=CIRCLE('',#16140,15.);
#6068=CIRCLE('',#16142,14.);
#6069=CIRCLE('',#16144,14.);
#6070=CIRCLE('',#16146,12.5);
#6071=CIRCLE('',#16148,12.5);
#6072=CIRCLE('',#16150,12.);
#6792=VERTEX_POINT('',#25743);
#6793=VERTEX_POINT('',#25744);
#6794=VERTEX_POINT('',#25746);
#6795=VERTEX_POINT('',#25750);
#6796=VERTEX_POINT('',#25757);
#6797=VERTEX_POINT('',#25758);
#6798=VERTEX_POINT('',#25760);
#6799=VERTEX_POINT('',#25764);
#6800=VERTEX_POINT('',#25772);
#6801=VERTEX_POINT('',#25776);
#6802=VERTEX_POINT('',#25782);
#6803=VERTEX_POINT('',#25784);
#6804=VERTEX_POINT('',#25786);
#6805=VERTEX_POINT('',#25788);
#6806=VERTEX_POINT('',#25794);
#6807=VERTEX_POINT('',#25798);
#6808=VERTEX_POINT('',#25802);
#6809=VERTEX_POINT('',#25804);
#6810=VERTEX_POINT('',#25808);
#6811=VERTEX_POINT('',#25809);
#6812=VERTEX_POINT('',#25811);
#6813=VERTEX_POINT('',#25815);
#6814=VERTEX_POINT('',#25822);
#6815=VERTEX_POINT('',#25823);
#6816=VERTEX_POINT('',#25825);
#6817=VERTEX_POINT('',#25829);
#6818=VERTEX_POINT('',#25837);
#6819=VERTEX_POINT('',#25841);
#6820=VERTEX_POINT('',#25847);
#6821=VERTEX_POINT('',#25849);
#6822=VERTEX_POINT('',#25851);
#6823=VERTEX_POINT('',#25853);
#6824=VERTEX_POINT('',#25859);
#6825=VERTEX_POINT('',#25863);
#6826=VERTEX_POINT('',#25867);
#6827=VERTEX_POINT('',#25869);
#6828=VERTEX_POINT('',#25873);
#6829=VERTEX_POINT('',#25874);
#6830=VERTEX_POINT('',#25876);
#6831=VERTEX_POINT('',#25880);
#6832=VERTEX_POINT('',#25887);
#6833=VERTEX_POINT('',#25888);
#6834=VERTEX_POINT('',#25890);
#6835=VERTEX_POINT('',#25894);
#6836=VERTEX_POINT('',#25902);
#6837=VERTEX_POINT('',#25906);
#6838=VERTEX_POINT('',#25912);
#6839=VERTEX_POINT('',#25914);
#6840=VERTEX_POINT('',#25916);
#6841=VERTEX_POINT('',#25918);
#6842=VERTEX_POINT('',#25924);
#6843=VERTEX_POINT('',#25928);
#6844=VERTEX_POINT('',#25932);
#6845=VERTEX_POINT('',#25934);
#6846=VERTEX_POINT('',#25938);
#6847=VERTEX_POINT('',#25939);
#6848=VERTEX_POINT('',#25941);
#6849=VERTEX_POINT('',#25945);
#6850=VERTEX_POINT('',#25952);
#6851=VERTEX_POINT('',#25953);
#6852=VERTEX_POINT('',#25955);
#6853=VERTEX_POINT('',#25959);
#6854=VERTEX_POINT('',#25967);
#6855=VERTEX_POINT('',#25971);
#6856=VERTEX_POINT('',#25977);
#6857=VERTEX_POINT('',#25979);
#6858=VERTEX_POINT('',#25981);
#6859=VERTEX_POINT('',#25983);
#6860=VERTEX_POINT('',#25989);
#6861=VERTEX_POINT('',#25993);
#6862=VERTEX_POINT('',#25997);
#6863=VERTEX_POINT('',#25999);
#6864=VERTEX_POINT('',#26003);
#6865=VERTEX_POINT('',#26004);
#6866=VERTEX_POINT('',#26008);
#6867=VERTEX_POINT('',#26010);
#6868=VERTEX_POINT('',#26016);
#6869=VERTEX_POINT('',#26020);
#6870=VERTEX_POINT('',#26022);
#6871=VERTEX_POINT('',#26024);
#6872=VERTEX_POINT('',#26026);
#6873=VERTEX_POINT('',#26032);
#6874=VERTEX_POINT('',#26033);
#6875=VERTEX_POINT('',#26035);
#6876=VERTEX_POINT('',#26039);
#6877=VERTEX_POINT('',#26046);
#6878=VERTEX_POINT('',#26053);
#6879=VERTEX_POINT('',#26057);
#6880=VERTEX_POINT('',#26059);
#6881=VERTEX_POINT('',#26061);
#6882=VERTEX_POINT('',#26065);
#6883=VERTEX_POINT('',#26067);
#6884=VERTEX_POINT('',#26071);
#6885=VERTEX_POINT('',#26077);
#6886=VERTEX_POINT('',#26079);
#6887=VERTEX_POINT('',#26081);
#6888=VERTEX_POINT('',#26083);
#6889=VERTEX_POINT('',#26085);
#6890=VERTEX_POINT('',#26087);
#6891=VERTEX_POINT('',#26089);
#6892=VERTEX_POINT('',#26091);
#6893=VERTEX_POINT('',#26093);
#6894=VERTEX_POINT('',#26095);
#6895=VERTEX_POINT('',#26097);
#6896=VERTEX_POINT('',#26099);
#6897=VERTEX_POINT('',#26101);
#6898=VERTEX_POINT('',#26103);
#6899=VERTEX_POINT('',#26105);
#6900=VERTEX_POINT('',#26112);
#6901=VERTEX_POINT('',#26114);
#6902=VERTEX_POINT('',#26116);
#6903=VERTEX_POINT('',#26118);
#6904=VERTEX_POINT('',#26120);
#6905=VERTEX_POINT('',#26122);
#6906=VERTEX_POINT('',#26124);
#6907=VERTEX_POINT('',#26126);
#6908=VERTEX_POINT('',#26128);
#6909=VERTEX_POINT('',#26130);
#6910=VERTEX_POINT('',#26132);
#6911=VERTEX_POINT('',#26134);
#6912=VERTEX_POINT('',#26136);
#6913=VERTEX_POINT('',#26138);
#6914=VERTEX_POINT('',#26140);
#6915=VERTEX_POINT('',#26142);
#6916=VERTEX_POINT('',#26144);
#6917=VERTEX_POINT('',#26146);
#6918=VERTEX_POINT('',#26150);
#6919=VERTEX_POINT('',#26157);
#6920=VERTEX_POINT('',#26161);
#6921=VERTEX_POINT('',#26168);
#6922=VERTEX_POINT('',#26172);
#6923=VERTEX_POINT('',#26178);
#6924=VERTEX_POINT('',#26180);
#6925=VERTEX_POINT('',#26182);
#6926=VERTEX_POINT('',#26186);
#6927=VERTEX_POINT('',#26190);
#6928=VERTEX_POINT('',#26194);
#6929=VERTEX_POINT('',#26196);
#6930=VERTEX_POINT('',#26200);
#6931=VERTEX_POINT('',#26201);
#6932=VERTEX_POINT('',#26211);
#6933=VERTEX_POINT('',#26215);
#6934=VERTEX_POINT('',#26222);
#6935=VERTEX_POINT('',#26226);
#6936=VERTEX_POINT('',#26232);
#6937=VERTEX_POINT('',#26234);
#6938=VERTEX_POINT('',#26236);
#6939=VERTEX_POINT('',#26238);
#6940=VERTEX_POINT('',#26244);
#6941=VERTEX_POINT('',#26248);
#6942=VERTEX_POINT('',#26252);
#6943=VERTEX_POINT('',#26254);
#6944=VERTEX_POINT('',#26258);
#6945=VERTEX_POINT('',#26259);
#6946=VERTEX_POINT('',#26261);
#6947=VERTEX_POINT('',#26263);
#6948=VERTEX_POINT('',#26267);
#6949=VERTEX_POINT('',#26269);
#6950=VERTEX_POINT('',#26273);
#6951=VERTEX_POINT('',#26274);
#6952=VERTEX_POINT('',#26276);
#6953=VERTEX_POINT('',#26278);
#6954=VERTEX_POINT('',#26282);
#6955=VERTEX_POINT('',#26284);
#6956=VERTEX_POINT('',#26288);
#6957=VERTEX_POINT('',#26289);
#6958=VERTEX_POINT('',#26291);
#6959=VERTEX_POINT('',#26293);
#6960=VERTEX_POINT('',#26297);
#6961=VERTEX_POINT('',#26299);
#6962=VERTEX_POINT('',#26303);
#6963=VERTEX_POINT('',#26304);
#6964=VERTEX_POINT('',#26306);
#6965=VERTEX_POINT('',#26308);
#6966=VERTEX_POINT('',#26312);
#6967=VERTEX_POINT('',#26314);
#6968=VERTEX_POINT('',#26318);
#6969=VERTEX_POINT('',#26319);
#6970=VERTEX_POINT('',#26321);
#6971=VERTEX_POINT('',#26323);
#6972=VERTEX_POINT('',#26327);
#6973=VERTEX_POINT('',#26329);
#6974=VERTEX_POINT('',#26362);
#6975=VERTEX_POINT('',#26363);
#6976=VERTEX_POINT('',#26373);
#6977=VERTEX_POINT('',#26377);
#6978=VERTEX_POINT('',#26384);
#6979=VERTEX_POINT('',#26388);
#6980=VERTEX_POINT('',#26395);
#6981=VERTEX_POINT('',#26403);
#6982=VERTEX_POINT('',#26409);
#6983=VERTEX_POINT('',#26410);
#6984=VERTEX_POINT('',#26420);
#6985=VERTEX_POINT('',#26424);
#6986=VERTEX_POINT('',#26431);
#6987=VERTEX_POINT('',#26435);
#6988=VERTEX_POINT('',#26442);
#6989=VERTEX_POINT('',#26450);
#6990=VERTEX_POINT('',#26456);
#6991=VERTEX_POINT('',#26457);
#6992=VERTEX_POINT('',#26467);
#6993=VERTEX_POINT('',#26471);
#6994=VERTEX_POINT('',#26478);
#6995=VERTEX_POINT('',#26482);
#6996=VERTEX_POINT('',#26489);
#6997=VERTEX_POINT('',#26497);
#6998=VERTEX_POINT('',#26503);
#6999=VERTEX_POINT('',#26504);
#7000=VERTEX_POINT('',#26514);
#7001=VERTEX_POINT('',#26518);
#7002=VERTEX_POINT('',#26525);
#7003=VERTEX_POINT('',#26529);
#7004=VERTEX_POINT('',#26536);
#7005=VERTEX_POINT('',#26544);
#7006=VERTEX_POINT('',#26550);
#7007=VERTEX_POINT('',#26551);
#7008=VERTEX_POINT('',#26561);
#7009=VERTEX_POINT('',#26565);
#7010=VERTEX_POINT('',#26572);
#7011=VERTEX_POINT('',#26576);
#7012=VERTEX_POINT('',#26585);
#7013=VERTEX_POINT('',#26591);
#7014=VERTEX_POINT('',#26595);
#7015=VERTEX_POINT('',#26601);
#7016=VERTEX_POINT('',#26602);
#7017=VERTEX_POINT('',#26604);
#7018=VERTEX_POINT('',#26606);
#7019=VERTEX_POINT('',#26610);
#7020=VERTEX_POINT('',#26612);
#7021=VERTEX_POINT('',#26616);
#7022=VERTEX_POINT('',#26623);
#7023=VERTEX_POINT('',#26627);
#7024=VERTEX_POINT('',#26634);
#7025=VERTEX_POINT('',#26638);
#7026=VERTEX_POINT('',#26647);
#7027=VERTEX_POINT('',#26655);
#7028=VERTEX_POINT('',#26657);
#7029=VERTEX_POINT('',#26661);
#7030=VERTEX_POINT('',#26675);
#7031=VERTEX_POINT('',#26680);
#7032=VERTEX_POINT('',#26681);
#7033=VERTEX_POINT('',#26683);
#7034=VERTEX_POINT('',#26685);
#7035=VERTEX_POINT('',#26689);
#7036=VERTEX_POINT('',#26691);
#7037=VERTEX_POINT('',#26695);
#7038=VERTEX_POINT('',#26697);
#7039=VERTEX_POINT('',#26721);
#7040=VERTEX_POINT('',#26724);
#7041=VERTEX_POINT('',#26728);
#7042=VERTEX_POINT('',#26731);
#7043=VERTEX_POINT('',#26735);
#7044=VERTEX_POINT('',#26738);
#7045=VERTEX_POINT('',#26742);
#8497=EDGE_CURVE('',#6792,#6793,#3846,.T.);
#8498=EDGE_CURVE('',#6793,#6794,#338,.T.);
#8499=EDGE_CURVE('',#6794,#6795,#3847,.T.);
#8500=EDGE_CURVE('',#6795,#6792,#1162,.T.);
#8501=EDGE_CURVE('',#6796,#6797,#3848,.T.);
#8502=EDGE_CURVE('',#6797,#6798,#339,.T.);
#8503=EDGE_CURVE('',#6798,#6799,#3849,.T.);
#8504=EDGE_CURVE('',#6799,#6796,#1163,.T.);
#8505=EDGE_CURVE('',#6795,#6796,#6007,.T.);
#8506=EDGE_CURVE('',#6799,#6800,#340,.T.);
#8507=EDGE_CURVE('',#6800,#6801,#6008,.T.);
#8508=EDGE_CURVE('',#6801,#6792,#341,.T.);
#8509=EDGE_CURVE('',#6801,#6802,#3850,.T.);
#8510=EDGE_CURVE('',#6803,#6802,#3851,.T.);
#8511=EDGE_CURVE('',#6804,#6803,#3852,.F.);
#8512=EDGE_CURVE('',#6805,#6804,#3853,.T.);
#8513=EDGE_CURVE('',#6793,#6805,#342,.T.);
#8514=EDGE_CURVE('',#6806,#6800,#3854,.T.);
#8515=EDGE_CURVE('',#6802,#6806,#3855,.T.);
#8516=EDGE_CURVE('',#6807,#6798,#343,.T.);
#8517=EDGE_CURVE('',#6808,#6807,#3856,.T.);
#8518=EDGE_CURVE('',#6809,#6808,#3857,.F.);
#8519=EDGE_CURVE('',#6809,#6806,#3858,.T.);
#8520=EDGE_CURVE('',#6810,#6811,#3859,.T.);
#8521=EDGE_CURVE('',#6811,#6812,#344,.T.);
#8522=EDGE_CURVE('',#6812,#6813,#3860,.T.);
#8523=EDGE_CURVE('',#6813,#6810,#1164,.T.);
#8524=EDGE_CURVE('',#6814,#6815,#3861,.T.);
#8525=EDGE_CURVE('',#6815,#6816,#345,.T.);
#8526=EDGE_CURVE('',#6816,#6817,#3862,.T.);
#8527=EDGE_CURVE('',#6817,#6814,#1165,.T.);
#8528=EDGE_CURVE('',#6813,#6814,#6009,.T.);
#8529=EDGE_CURVE('',#6817,#6818,#346,.T.);
#8530=EDGE_CURVE('',#6818,#6819,#6010,.T.);
#8531=EDGE_CURVE('',#6819,#6810,#347,.T.);
#8532=EDGE_CURVE('',#6819,#6820,#3863,.T.);
#8533=EDGE_CURVE('',#6821,#6820,#3864,.T.);
#8534=EDGE_CURVE('',#6822,#6821,#3865,.F.);
#8535=EDGE_CURVE('',#6823,#6822,#3866,.T.);
#8536=EDGE_CURVE('',#6811,#6823,#348,.T.);
#8537=EDGE_CURVE('',#6824,#6818,#3867,.T.);
#8538=EDGE_CURVE('',#6820,#6824,#3868,.T.);
#8539=EDGE_CURVE('',#6825,#6816,#349,.T.);
#8540=EDGE_CURVE('',#6826,#6825,#3869,.T.);
#8541=EDGE_CURVE('',#6827,#6826,#3870,.F.);
#8542=EDGE_CURVE('',#6827,#6824,#3871,.T.);
#8543=EDGE_CURVE('',#6828,#6829,#3872,.T.);
#8544=EDGE_CURVE('',#6829,#6830,#350,.T.);
#8545=EDGE_CURVE('',#6830,#6831,#3873,.T.);
#8546=EDGE_CURVE('',#6831,#6828,#1166,.T.);
#8547=EDGE_CURVE('',#6832,#6833,#3874,.T.);
#8548=EDGE_CURVE('',#6833,#6834,#351,.T.);
#8549=EDGE_CURVE('',#6834,#6835,#3875,.T.);
#8550=EDGE_CURVE('',#6835,#6832,#1167,.T.);
#8551=EDGE_CURVE('',#6831,#6832,#6011,.T.);
#8552=EDGE_CURVE('',#6835,#6836,#352,.T.);
#8553=EDGE_CURVE('',#6836,#6837,#6012,.T.);
#8554=EDGE_CURVE('',#6837,#6828,#353,.T.);
#8555=EDGE_CURVE('',#6837,#6838,#3876,.T.);
#8556=EDGE_CURVE('',#6839,#6838,#3877,.T.);
#8557=EDGE_CURVE('',#6840,#6839,#3878,.F.);
#8558=EDGE_CURVE('',#6841,#6840,#3879,.T.);
#8559=EDGE_CURVE('',#6829,#6841,#354,.T.);
#8560=EDGE_CURVE('',#6842,#6836,#3880,.T.);
#8561=EDGE_CURVE('',#6838,#6842,#3881,.T.);
#8562=EDGE_CURVE('',#6843,#6834,#355,.T.);
#8563=EDGE_CURVE('',#6844,#6843,#3882,.T.);
#8564=EDGE_CURVE('',#6845,#6844,#3883,.F.);
#8565=EDGE_CURVE('',#6845,#6842,#3884,.T.);
#8566=EDGE_CURVE('',#6846,#6847,#3885,.T.);
#8567=EDGE_CURVE('',#6847,#6848,#356,.T.);
#8568=EDGE_CURVE('',#6848,#6849,#3886,.T.);
#8569=EDGE_CURVE('',#6849,#6846,#1168,.T.);
#8570=EDGE_CURVE('',#6850,#6851,#3887,.T.);
#8571=EDGE_CURVE('',#6851,#6852,#357,.T.);
#8572=EDGE_CURVE('',#6852,#6853,#3888,.T.);
#8573=EDGE_CURVE('',#6853,#6850,#1169,.T.);
#8574=EDGE_CURVE('',#6849,#6850,#6013,.T.);
#8575=EDGE_CURVE('',#6853,#6854,#358,.T.);
#8576=EDGE_CURVE('',#6854,#6855,#6014,.T.);
#8577=EDGE_CURVE('',#6855,#6846,#359,.T.);
#8578=EDGE_CURVE('',#6855,#6856,#3889,.T.);
#8579=EDGE_CURVE('',#6857,#6856,#3890,.T.);
#8580=EDGE_CURVE('',#6858,#6857,#3891,.F.);
#8581=EDGE_CURVE('',#6859,#6858,#3892,.T.);
#8582=EDGE_CURVE('',#6847,#6859,#360,.T.);
#8583=EDGE_CURVE('',#6860,#6854,#3893,.T.);
#8584=EDGE_CURVE('',#6856,#6860,#3894,.T.);
#8585=EDGE_CURVE('',#6861,#6852,#361,.T.);
#8586=EDGE_CURVE('',#6862,#6861,#3895,.T.);
#8587=EDGE_CURVE('',#6863,#6862,#3896,.F.);
#8588=EDGE_CURVE('',#6863,#6860,#3897,.T.);
#8589=EDGE_CURVE('',#6864,#6865,#362,.T.);
#8590=EDGE_CURVE('',#6865,#6866,#3898,.T.);
#8591=EDGE_CURVE('',#6866,#6867,#363,.F.);
#8592=EDGE_CURVE('',#6867,#6864,#3899,.T.);
#8593=EDGE_CURVE('',#6868,#6867,#364,.F.);
#8594=EDGE_CURVE('',#6868,#6869,#3900,.T.);
#8595=EDGE_CURVE('',#6870,#6869,#3901,.T.);
#8596=EDGE_CURVE('',#6871,#6870,#3902,.F.);
#8597=EDGE_CURVE('',#6872,#6871,#3903,.T.);
#8598=EDGE_CURVE('',#6864,#6872,#365,.T.);
#8599=EDGE_CURVE('',#6873,#6874,#3904,.T.);
#8600=EDGE_CURVE('',#6874,#6875,#366,.T.);
#8601=EDGE_CURVE('',#6875,#6876,#3905,.T.);
#8602=EDGE_CURVE('',#6876,#6873,#1170,.T.);
#8603=EDGE_CURVE('',#6877,#6868,#6015,.T.);
#8604=EDGE_CURVE('',#6866,#6873,#6016,.T.);
#8605=EDGE_CURVE('',#6876,#6877,#367,.T.);
#8606=EDGE_CURVE('',#6878,#6875,#368,.T.);
#8607=EDGE_CURVE('',#6879,#6878,#3906,.T.);
#8608=EDGE_CURVE('',#6880,#6879,#3907,.F.);
#8609=EDGE_CURVE('',#6880,#6881,#3908,.T.);
#8610=EDGE_CURVE('',#6881,#6877,#3909,.T.);
#8611=EDGE_CURVE('',#6882,#6874,#6017,.T.);
#8612=EDGE_CURVE('',#6883,#6882,#369,.T.);
#8613=EDGE_CURVE('',#6883,#6884,#370,.T.);
#8614=EDGE_CURVE('',#6884,#6878,#6018,.T.);
#8615=EDGE_CURVE('',#6885,#6885,#6019,.T.);
#8616=EDGE_CURVE('',#6885,#6886,#3910,.T.);
#8617=EDGE_CURVE('',#6887,#6886,#6020,.T.);
#8618=EDGE_CURVE('',#6888,#6887,#3911,.T.);
#8619=EDGE_CURVE('',#6888,#6889,#6021,.T.);
#8620=EDGE_CURVE('',#6890,#6889,#3912,.T.);
#8621=EDGE_CURVE('',#6891,#6890,#6022,.T.);
#8622=EDGE_CURVE('',#6892,#6891,#3913,.T.);
#8623=EDGE_CURVE('',#6892,#6893,#6023,.T.);
#8624=EDGE_CURVE('',#6894,#6893,#3914,.T.);
#8625=EDGE_CURVE('',#6895,#6894,#6024,.T.);
#8626=EDGE_CURVE('',#6896,#6895,#3915,.T.);
#8627=EDGE_CURVE('',#6896,#6897,#6025,.T.);
#8628=EDGE_CURVE('',#6898,#6897,#3916,.T.);
#8629=EDGE_CURVE('',#6899,#6898,#6026,.T.);
#8630=EDGE_CURVE('',#6882,#6899,#3917,.T.);
#8631=EDGE_CURVE('',#6865,#6851,#6027,.T.);
#8632=EDGE_CURVE('',#6848,#6833,#6028,.T.);
#8633=EDGE_CURVE('',#6830,#6815,#6029,.T.);
#8634=EDGE_CURVE('',#6812,#6797,#6030,.T.);
#8635=EDGE_CURVE('',#6794,#6900,#6031,.T.);
#8636=EDGE_CURVE('',#6901,#6900,#3918,.T.);
#8637=EDGE_CURVE('',#6902,#6901,#6032,.T.);
#8638=EDGE_CURVE('',#6903,#6902,#3919,.T.);
#8639=EDGE_CURVE('',#6903,#6904,#6033,.T.);
#8640=EDGE_CURVE('',#6905,#6904,#3920,.T.);
#8641=EDGE_CURVE('',#6906,#6905,#6034,.T.);
#8642=EDGE_CURVE('',#6907,#6906,#3921,.T.);
#8643=EDGE_CURVE('',#6907,#6908,#6035,.T.);
#8644=EDGE_CURVE('',#6909,#6908,#3922,.T.);
#8645=EDGE_CURVE('',#6910,#6909,#6036,.T.);
#8646=EDGE_CURVE('',#6911,#6910,#3923,.T.);
#8647=EDGE_CURVE('',#6911,#6912,#6037,.T.);
#8648=EDGE_CURVE('',#6913,#6912,#3924,.T.);
#8649=EDGE_CURVE('',#6914,#6913,#6038,.T.);
#8650=EDGE_CURVE('',#6915,#6914,#3925,.T.);
#8651=EDGE_CURVE('',#6915,#6916,#6039,.T.);
#8652=EDGE_CURVE('',#6917,#6916,#3926,.T.);
#8653=EDGE_CURVE('',#6886,#6917,#6040,.T.);
#8654=EDGE_CURVE('',#6918,#6883,#3927,.T.);
#8655=EDGE_CURVE('',#6899,#6918,#1171,.T.);
#8656=EDGE_CURVE('',#6897,#6919,#371,.T.);
#8657=EDGE_CURVE('',#6919,#6920,#3928,.T.);
#8658=EDGE_CURVE('',#6920,#6898,#1172,.T.);
#8659=EDGE_CURVE('',#6920,#6921,#372,.T.);
#8660=EDGE_CURVE('',#6921,#6922,#6041,.T.);
#8661=EDGE_CURVE('',#6922,#6918,#373,.T.);
#8662=EDGE_CURVE('',#6922,#6923,#3929,.T.);
#8663=EDGE_CURVE('',#6924,#6923,#3930,.T.);
#8664=EDGE_CURVE('',#6925,#6924,#3931,.F.);
#8665=EDGE_CURVE('',#6884,#6925,#3932,.T.);
#8666=EDGE_CURVE('',#6926,#6921,#3933,.T.);
#8667=EDGE_CURVE('',#6923,#6926,#3934,.T.);
#8668=EDGE_CURVE('',#6927,#6919,#374,.T.);
#8669=EDGE_CURVE('',#6928,#6927,#3935,.T.);
#8670=EDGE_CURVE('',#6929,#6928,#3936,.F.);
#8671=EDGE_CURVE('',#6929,#6926,#3937,.T.);
#8672=EDGE_CURVE('',#6930,#6931,#3938,.T.);
#8673=EDGE_CURVE('',#6931,#6896,#375,.T.);
#8674=EDGE_CURVE('',#6895,#6930,#1173,.T.);
#8675=EDGE_CURVE('',#6893,#6932,#376,.T.);
#8676=EDGE_CURVE('',#6932,#6933,#3939,.T.);
#8677=EDGE_CURVE('',#6933,#6894,#1174,.T.);
#8678=EDGE_CURVE('',#6933,#6934,#377,.T.);
#8679=EDGE_CURVE('',#6934,#6935,#6042,.T.);
#8680=EDGE_CURVE('',#6935,#6930,#378,.T.);
#8681=EDGE_CURVE('',#6935,#6936,#3940,.T.);
#8682=EDGE_CURVE('',#6937,#6936,#3941,.T.);
#8683=EDGE_CURVE('',#6938,#6937,#3942,.F.);
#8684=EDGE_CURVE('',#6939,#6938,#3943,.T.);
#8685=EDGE_CURVE('',#6931,#6939,#379,.T.);
#8686=EDGE_CURVE('',#6940,#6934,#3944,.T.);
#8687=EDGE_CURVE('',#6936,#6940,#3945,.T.);
#8688=EDGE_CURVE('',#6941,#6932,#380,.T.);
#8689=EDGE_CURVE('',#6942,#6941,#3946,.T.);
#8690=EDGE_CURVE('',#6943,#6942,#3947,.F.);
#8691=EDGE_CURVE('',#6943,#6940,#3948,.T.);
#8692=EDGE_CURVE('',#6944,#6945,#3949,.F.);
#8693=EDGE_CURVE('',#6945,#6946,#3950,.T.);
#8694=EDGE_CURVE('',#6946,#6947,#3951,.F.);
#8695=EDGE_CURVE('',#6947,#6944,#3952,.T.);
#8696=EDGE_CURVE('',#6945,#6948,#3953,.T.);
#8697=EDGE_CURVE('',#6948,#6949,#3954,.T.);
#8698=EDGE_CURVE('',#6946,#6949,#3955,.T.);
#8699=EDGE_CURVE('',#6950,#6951,#3956,.F.);
#8700=EDGE_CURVE('',#6951,#6952,#3957,.T.);
#8701=EDGE_CURVE('',#6952,#6953,#3958,.F.);
#8702=EDGE_CURVE('',#6953,#6950,#3959,.T.);
#8703=EDGE_CURVE('',#6951,#6954,#3960,.T.);
#8704=EDGE_CURVE('',#6954,#6955,#3961,.T.);
#8705=EDGE_CURVE('',#6952,#6955,#3962,.T.);
#8706=EDGE_CURVE('',#6956,#6957,#3963,.F.);
#8707=EDGE_CURVE('',#6957,#6958,#3964,.T.);
#8708=EDGE_CURVE('',#6958,#6959,#3965,.F.);
#8709=EDGE_CURVE('',#6959,#6956,#3966,.T.);
#8710=EDGE_CURVE('',#6957,#6960,#3967,.T.);
#8711=EDGE_CURVE('',#6960,#6961,#3968,.T.);
#8712=EDGE_CURVE('',#6958,#6961,#3969,.T.);
#8713=EDGE_CURVE('',#6962,#6963,#3970,.F.);
#8714=EDGE_CURVE('',#6963,#6964,#3971,.T.);
#8715=EDGE_CURVE('',#6964,#6965,#3972,.F.);
#8716=EDGE_CURVE('',#6965,#6962,#3973,.T.);
#8717=EDGE_CURVE('',#6963,#6966,#3974,.T.);
#8718=EDGE_CURVE('',#6966,#6967,#3975,.T.);
#8719=EDGE_CURVE('',#6964,#6967,#3976,.T.);
#8720=EDGE_CURVE('',#6968,#6969,#3977,.F.);
#8721=EDGE_CURVE('',#6969,#6970,#3978,.T.);
#8722=EDGE_CURVE('',#6970,#6971,#3979,.F.);
#8723=EDGE_CURVE('',#6971,#6968,#3980,.T.);
#8724=EDGE_CURVE('',#6969,#6972,#3981,.T.);
#8725=EDGE_CURVE('',#6972,#6973,#3982,.T.);
#8726=EDGE_CURVE('',#6970,#6973,#3983,.T.);
#8727=EDGE_CURVE('',#6937,#6943,#3984,.T.);
#8728=EDGE_CURVE('',#6942,#6938,#3985,.T.);
#8729=EDGE_CURVE('',#6924,#6929,#3986,.T.);
#8730=EDGE_CURVE('',#6928,#6925,#3987,.T.);
#8731=EDGE_CURVE('',#6870,#6880,#3988,.T.);
#8732=EDGE_CURVE('',#6879,#6871,#3989,.T.);
#8733=EDGE_CURVE('',#6869,#6881,#3990,.T.);
#8734=EDGE_CURVE('',#6857,#6863,#3991,.T.);
#8735=EDGE_CURVE('',#6862,#6858,#3992,.T.);
#8736=EDGE_CURVE('',#6839,#6845,#3993,.T.);
#8737=EDGE_CURVE('',#6844,#6840,#3994,.T.);
#8738=EDGE_CURVE('',#6821,#6827,#3995,.T.);
#8739=EDGE_CURVE('',#6826,#6822,#3996,.T.);
#8740=EDGE_CURVE('',#6803,#6809,#3997,.T.);
#8741=EDGE_CURVE('',#6808,#6804,#3998,.T.);
#8742=EDGE_CURVE('',#6974,#6975,#3999,.T.);
#8743=EDGE_CURVE('',#6975,#6892,#381,.T.);
#8744=EDGE_CURVE('',#6891,#6974,#1175,.T.);
#8745=EDGE_CURVE('',#6889,#6976,#382,.T.);
#8746=EDGE_CURVE('',#6976,#6977,#4000,.T.);
#8747=EDGE_CURVE('',#6977,#6890,#1176,.T.);
#8748=EDGE_CURVE('',#6977,#6978,#383,.T.);
#8749=EDGE_CURVE('',#6978,#6979,#6043,.T.);
#8750=EDGE_CURVE('',#6979,#6974,#384,.T.);
#8751=EDGE_CURVE('',#6979,#6972,#4001,.T.);
#8752=EDGE_CURVE('',#6980,#6968,#4002,.T.);
#8753=EDGE_CURVE('',#6975,#6980,#385,.T.);
#8754=EDGE_CURVE('',#6973,#6978,#4003,.T.);
#8755=EDGE_CURVE('',#6981,#6976,#386,.T.);
#8756=EDGE_CURVE('',#6971,#6981,#4004,.T.);
#8757=EDGE_CURVE('',#6982,#6983,#4005,.T.);
#8758=EDGE_CURVE('',#6983,#6888,#387,.T.);
#8759=EDGE_CURVE('',#6887,#6982,#1177,.T.);
#8760=EDGE_CURVE('',#6916,#6984,#388,.T.);
#8761=EDGE_CURVE('',#6984,#6985,#4006,.T.);
#8762=EDGE_CURVE('',#6985,#6917,#1178,.T.);
#8763=EDGE_CURVE('',#6985,#6986,#389,.T.);
#8764=EDGE_CURVE('',#6986,#6987,#6044,.T.);
#8765=EDGE_CURVE('',#6987,#6982,#390,.T.);
#8766=EDGE_CURVE('',#6987,#6966,#4007,.T.);
#8767=EDGE_CURVE('',#6988,#6962,#4008,.T.);
#8768=EDGE_CURVE('',#6983,#6988,#391,.T.);
#8769=EDGE_CURVE('',#6967,#6986,#4009,.T.);
#8770=EDGE_CURVE('',#6989,#6984,#392,.T.);
#8771=EDGE_CURVE('',#6965,#6989,#4010,.T.);
#8772=EDGE_CURVE('',#6990,#6991,#4011,.T.);
#8773=EDGE_CURVE('',#6991,#6915,#393,.T.);
#8774=EDGE_CURVE('',#6914,#6990,#1179,.T.);
#8775=EDGE_CURVE('',#6912,#6992,#394,.T.);
#8776=EDGE_CURVE('',#6992,#6993,#4012,.T.);
#8777=EDGE_CURVE('',#6993,#6913,#1180,.T.);
#8778=EDGE_CURVE('',#6993,#6994,#395,.T.);
#8779=EDGE_CURVE('',#6994,#6995,#6045,.T.);
#8780=EDGE_CURVE('',#6995,#6990,#396,.T.);
#8781=EDGE_CURVE('',#6995,#6960,#4013,.T.);
#8782=EDGE_CURVE('',#6996,#6956,#4014,.T.);
#8783=EDGE_CURVE('',#6991,#6996,#397,.T.);
#8784=EDGE_CURVE('',#6961,#6994,#4015,.T.);
#8785=EDGE_CURVE('',#6997,#6992,#398,.T.);
#8786=EDGE_CURVE('',#6959,#6997,#4016,.T.);
#8787=EDGE_CURVE('',#6998,#6999,#4017,.T.);
#8788=EDGE_CURVE('',#6999,#6911,#399,.T.);
#8789=EDGE_CURVE('',#6910,#6998,#1181,.T.);
#8790=EDGE_CURVE('',#6908,#7000,#400,.T.);
#8791=EDGE_CURVE('',#7000,#7001,#4018,.T.);
#8792=EDGE_CURVE('',#7001,#6909,#1182,.T.);
#8793=EDGE_CURVE('',#7001,#7002,#401,.T.);
#8794=EDGE_CURVE('',#7002,#7003,#6046,.T.);
#8795=EDGE_CURVE('',#7003,#6998,#402,.T.);
#8796=EDGE_CURVE('',#7003,#6954,#4019,.T.);
#8797=EDGE_CURVE('',#7004,#6950,#4020,.T.);
#8798=EDGE_CURVE('',#6999,#7004,#403,.T.);
#8799=EDGE_CURVE('',#6955,#7002,#4021,.T.);
#8800=EDGE_CURVE('',#7005,#7000,#404,.T.);
#8801=EDGE_CURVE('',#6953,#7005,#4022,.T.);
#8802=EDGE_CURVE('',#7006,#7007,#4023,.T.);
#8803=EDGE_CURVE('',#7007,#6907,#405,.T.);
#8804=EDGE_CURVE('',#6906,#7006,#1183,.T.);
#8805=EDGE_CURVE('',#6904,#7008,#406,.T.);
#8806=EDGE_CURVE('',#7008,#7009,#4024,.T.);
#8807=EDGE_CURVE('',#7009,#6905,#1184,.T.);
#8808=EDGE_CURVE('',#7009,#7010,#407,.T.);
#8809=EDGE_CURVE('',#7010,#7011,#6047,.T.);
#8810=EDGE_CURVE('',#7011,#7006,#408,.T.);
#8811=EDGE_CURVE('',#6949,#7010,#4025,.T.);
#8812=EDGE_CURVE('',#7011,#6948,#4026,.T.);
#8813=EDGE_CURVE('',#7012,#7008,#409,.T.);
#8814=EDGE_CURVE('',#6947,#7012,#4027,.T.);
#8815=EDGE_CURVE('',#7013,#6903,#410,.T.);
#8816=EDGE_CURVE('',#7013,#7014,#411,.T.);
#8817=EDGE_CURVE('',#7014,#7012,#6048,.T.);
#8818=EDGE_CURVE('',#7015,#7016,#4028,.F.);
#8819=EDGE_CURVE('',#7016,#7017,#4029,.T.);
#8820=EDGE_CURVE('',#7017,#7018,#4030,.F.);
#8821=EDGE_CURVE('',#7018,#7015,#4031,.T.);
#8822=EDGE_CURVE('',#7016,#7019,#4032,.T.);
#8823=EDGE_CURVE('',#7019,#7020,#4033,.T.);
#8824=EDGE_CURVE('',#7017,#7020,#4034,.T.);
#8825=EDGE_CURVE('',#7021,#7013,#4035,.T.);
#8826=EDGE_CURVE('',#6902,#7021,#1185,.T.);
#8827=EDGE_CURVE('',#6900,#7022,#412,.T.);
#8828=EDGE_CURVE('',#7022,#7023,#4036,.T.);
#8829=EDGE_CURVE('',#7023,#6901,#1186,.T.);
#8830=EDGE_CURVE('',#7023,#7024,#413,.T.);
#8831=EDGE_CURVE('',#7024,#7025,#6049,.T.);
#8832=EDGE_CURVE('',#7025,#7021,#414,.T.);
#8833=EDGE_CURVE('',#7020,#7024,#4037,.T.);
#8834=EDGE_CURVE('',#7025,#7019,#4038,.T.);
#8835=EDGE_CURVE('',#7026,#7022,#415,.T.);
#8836=EDGE_CURVE('',#7018,#7026,#4039,.T.);
#8837=EDGE_CURVE('',#6805,#7026,#6050,.T.);
#8838=EDGE_CURVE('',#7027,#7027,#6051,.T.);
#8839=EDGE_CURVE('',#7027,#7028,#4040,.T.);
#8840=EDGE_CURVE('',#7028,#7028,#6052,.T.);
#8841=EDGE_CURVE('',#7028,#7029,#4041,.T.);
#8842=EDGE_CURVE('',#7029,#7029,#6053,.T.);
#8843=EDGE_CURVE('',#7014,#7015,#4042,.T.);
#8844=EDGE_CURVE('',#6823,#6807,#6054,.T.);
#8845=EDGE_CURVE('',#6841,#6825,#6055,.T.);
#8846=EDGE_CURVE('',#6859,#6843,#6056,.T.);
#8847=EDGE_CURVE('',#6872,#6861,#6057,.T.);
#8848=EDGE_CURVE('',#6939,#6927,#6058,.T.);
#8849=EDGE_CURVE('',#6980,#6941,#6059,.T.);
#8850=EDGE_CURVE('',#6988,#6981,#6060,.T.);
#8851=EDGE_CURVE('',#6996,#6989,#6061,.T.);
#8852=EDGE_CURVE('',#7004,#6997,#6062,.T.);
#8853=EDGE_CURVE('',#7030,#7005,#6063,.T.);
#8854=EDGE_CURVE('',#7030,#6944,#4043,.T.);
#8855=EDGE_CURVE('',#7031,#7032,#6064,.T.);
#8856=EDGE_CURVE('',#7031,#7033,#4044,.T.);
#8857=EDGE_CURVE('',#7033,#7034,#4045,.T.);
#8858=EDGE_CURVE('',#7032,#7034,#4046,.T.);
#8859=EDGE_CURVE('',#7032,#7035,#4047,.T.);
#8860=EDGE_CURVE('',#7034,#7036,#4048,.T.);
#8861=EDGE_CURVE('',#7035,#7036,#4049,.T.);
#8862=EDGE_CURVE('',#7037,#7031,#4050,.T.);
#8863=EDGE_CURVE('',#7037,#7038,#4051,.T.);
#8864=EDGE_CURVE('',#7038,#7033,#4052,.T.);
#8865=EDGE_CURVE('',#7035,#7037,#6065,.T.);
#8866=EDGE_CURVE('',#7036,#7038,#4053,.T.);
#8867=EDGE_CURVE('',#7007,#7030,#416,.T.);
#8868=EDGE_CURVE('',#7039,#7039,#6066,.T.);
#8869=EDGE_CURVE('',#7040,#7040,#6067,.T.);
#8870=EDGE_CURVE('',#7040,#7039,#4054,.T.);
#8871=EDGE_CURVE('',#7041,#7041,#6068,.T.);
#8872=EDGE_CURVE('',#7042,#7042,#6069,.T.);
#8873=EDGE_CURVE('',#7042,#7041,#4055,.T.);
#8874=EDGE_CURVE('',#7043,#7043,#6070,.T.);
#8875=EDGE_CURVE('',#7044,#7044,#6071,.T.);
#8876=EDGE_CURVE('',#7044,#7043,#4056,.T.);
#8877=EDGE_CURVE('',#7045,#7045,#6072,.T.);
#8878=EDGE_CURVE('',#7045,#7044,#4057,.T.);
#11497=ORIENTED_EDGE('',*,*,#8497,.T.);
#11498=ORIENTED_EDGE('',*,*,#8498,.T.);
#11499=ORIENTED_EDGE('',*,*,#8499,.T.);
#11500=ORIENTED_EDGE('',*,*,#8500,.T.);
#11501=ORIENTED_EDGE('',*,*,#8501,.T.);
#11502=ORIENTED_EDGE('',*,*,#8502,.T.);
#11503=ORIENTED_EDGE('',*,*,#8503,.T.);
#11504=ORIENTED_EDGE('',*,*,#8504,.T.);
#11505=ORIENTED_EDGE('',*,*,#8505,.T.);
#11506=ORIENTED_EDGE('',*,*,#8504,.F.);
#11507=ORIENTED_EDGE('',*,*,#8506,.T.);
#11508=ORIENTED_EDGE('',*,*,#8507,.T.);
#11509=ORIENTED_EDGE('',*,*,#8508,.T.);
#11510=ORIENTED_EDGE('',*,*,#8500,.F.);
#11511=ORIENTED_EDGE('',*,*,#8497,.F.);
#11512=ORIENTED_EDGE('',*,*,#8508,.F.);
#11513=ORIENTED_EDGE('',*,*,#8509,.T.);
#11514=ORIENTED_EDGE('',*,*,#8510,.F.);
#11515=ORIENTED_EDGE('',*,*,#8511,.F.);
#11516=ORIENTED_EDGE('',*,*,#8512,.F.);
#11517=ORIENTED_EDGE('',*,*,#8513,.F.);
#11518=ORIENTED_EDGE('',*,*,#8507,.F.);
#11519=ORIENTED_EDGE('',*,*,#8514,.F.);
#11520=ORIENTED_EDGE('',*,*,#8515,.F.);
#11521=ORIENTED_EDGE('',*,*,#8509,.F.);
#11522=ORIENTED_EDGE('',*,*,#8503,.F.);
#11523=ORIENTED_EDGE('',*,*,#8516,.F.);
#11524=ORIENTED_EDGE('',*,*,#8517,.F.);
#11525=ORIENTED_EDGE('',*,*,#8518,.F.);
#11526=ORIENTED_EDGE('',*,*,#8519,.T.);
#11527=ORIENTED_EDGE('',*,*,#8514,.T.);
#11528=ORIENTED_EDGE('',*,*,#8506,.F.);
#11529=ORIENTED_EDGE('',*,*,#8520,.T.);
#11530=ORIENTED_EDGE('',*,*,#8521,.T.);
#11531=ORIENTED_EDGE('',*,*,#8522,.T.);
#11532=ORIENTED_EDGE('',*,*,#8523,.T.);
#11533=ORIENTED_EDGE('',*,*,#8524,.T.);
#11534=ORIENTED_EDGE('',*,*,#8525,.T.);
#11535=ORIENTED_EDGE('',*,*,#8526,.T.);
#11536=ORIENTED_EDGE('',*,*,#8527,.T.);
#11537=ORIENTED_EDGE('',*,*,#8528,.T.);
#11538=ORIENTED_EDGE('',*,*,#8527,.F.);
#11539=ORIENTED_EDGE('',*,*,#8529,.T.);
#11540=ORIENTED_EDGE('',*,*,#8530,.T.);
#11541=ORIENTED_EDGE('',*,*,#8531,.T.);
#11542=ORIENTED_EDGE('',*,*,#8523,.F.);
#11543=ORIENTED_EDGE('',*,*,#8520,.F.);
#11544=ORIENTED_EDGE('',*,*,#8531,.F.);
#11545=ORIENTED_EDGE('',*,*,#8532,.T.);
#11546=ORIENTED_EDGE('',*,*,#8533,.F.);
#11547=ORIENTED_EDGE('',*,*,#8534,.F.);
#11548=ORIENTED_EDGE('',*,*,#8535,.F.);
#11549=ORIENTED_EDGE('',*,*,#8536,.F.);
#11550=ORIENTED_EDGE('',*,*,#8530,.F.);
#11551=ORIENTED_EDGE('',*,*,#8537,.F.);
#11552=ORIENTED_EDGE('',*,*,#8538,.F.);
#11553=ORIENTED_EDGE('',*,*,#8532,.F.);
#11554=ORIENTED_EDGE('',*,*,#8526,.F.);
#11555=ORIENTED_EDGE('',*,*,#8539,.F.);
#11556=ORIENTED_EDGE('',*,*,#8540,.F.);
#11557=ORIENTED_EDGE('',*,*,#8541,.F.);
#11558=ORIENTED_EDGE('',*,*,#8542,.T.);
#11559=ORIENTED_EDGE('',*,*,#8537,.T.);
#11560=ORIENTED_EDGE('',*,*,#8529,.F.);
#11561=ORIENTED_EDGE('',*,*,#8543,.T.);
#11562=ORIENTED_EDGE('',*,*,#8544,.T.);
#11563=ORIENTED_EDGE('',*,*,#8545,.T.);
#11564=ORIENTED_EDGE('',*,*,#8546,.T.);
#11565=ORIENTED_EDGE('',*,*,#8547,.T.);
#11566=ORIENTED_EDGE('',*,*,#8548,.T.);
#11567=ORIENTED_EDGE('',*,*,#8549,.T.);
#11568=ORIENTED_EDGE('',*,*,#8550,.T.);
#11569=ORIENTED_EDGE('',*,*,#8551,.T.);
#11570=ORIENTED_EDGE('',*,*,#8550,.F.);
#11571=ORIENTED_EDGE('',*,*,#8552,.T.);
#11572=ORIENTED_EDGE('',*,*,#8553,.T.);
#11573=ORIENTED_EDGE('',*,*,#8554,.T.);
#11574=ORIENTED_EDGE('',*,*,#8546,.F.);
#11575=ORIENTED_EDGE('',*,*,#8543,.F.);
#11576=ORIENTED_EDGE('',*,*,#8554,.F.);
#11577=ORIENTED_EDGE('',*,*,#8555,.T.);
#11578=ORIENTED_EDGE('',*,*,#8556,.F.);
#11579=ORIENTED_EDGE('',*,*,#8557,.F.);
#11580=ORIENTED_EDGE('',*,*,#8558,.F.);
#11581=ORIENTED_EDGE('',*,*,#8559,.F.);
#11582=ORIENTED_EDGE('',*,*,#8553,.F.);
#11583=ORIENTED_EDGE('',*,*,#8560,.F.);
#11584=ORIENTED_EDGE('',*,*,#8561,.F.);
#11585=ORIENTED_EDGE('',*,*,#8555,.F.);
#11586=ORIENTED_EDGE('',*,*,#8549,.F.);
#11587=ORIENTED_EDGE('',*,*,#8562,.F.);
#11588=ORIENTED_EDGE('',*,*,#8563,.F.);
#11589=ORIENTED_EDGE('',*,*,#8564,.F.);
#11590=ORIENTED_EDGE('',*,*,#8565,.T.);
#11591=ORIENTED_EDGE('',*,*,#8560,.T.);
#11592=ORIENTED_EDGE('',*,*,#8552,.F.);
#11593=ORIENTED_EDGE('',*,*,#8566,.T.);
#11594=ORIENTED_EDGE('',*,*,#8567,.T.);
#11595=ORIENTED_EDGE('',*,*,#8568,.T.);
#11596=ORIENTED_EDGE('',*,*,#8569,.T.);
#11597=ORIENTED_EDGE('',*,*,#8570,.T.);
#11598=ORIENTED_EDGE('',*,*,#8571,.T.);
#11599=ORIENTED_EDGE('',*,*,#8572,.T.);
#11600=ORIENTED_EDGE('',*,*,#8573,.T.);
#11601=ORIENTED_EDGE('',*,*,#8574,.T.);
#11602=ORIENTED_EDGE('',*,*,#8573,.F.);
#11603=ORIENTED_EDGE('',*,*,#8575,.T.);
#11604=ORIENTED_EDGE('',*,*,#8576,.T.);
#11605=ORIENTED_EDGE('',*,*,#8577,.T.);
#11606=ORIENTED_EDGE('',*,*,#8569,.F.);
#11607=ORIENTED_EDGE('',*,*,#8566,.F.);
#11608=ORIENTED_EDGE('',*,*,#8577,.F.);
#11609=ORIENTED_EDGE('',*,*,#8578,.T.);
#11610=ORIENTED_EDGE('',*,*,#8579,.F.);
#11611=ORIENTED_EDGE('',*,*,#8580,.F.);
#11612=ORIENTED_EDGE('',*,*,#8581,.F.);
#11613=ORIENTED_EDGE('',*,*,#8582,.F.);
#11614=ORIENTED_EDGE('',*,*,#8576,.F.);
#11615=ORIENTED_EDGE('',*,*,#8583,.F.);
#11616=ORIENTED_EDGE('',*,*,#8584,.F.);
#11617=ORIENTED_EDGE('',*,*,#8578,.F.);
#11618=ORIENTED_EDGE('',*,*,#8572,.F.);
#11619=ORIENTED_EDGE('',*,*,#8585,.F.);
#11620=ORIENTED_EDGE('',*,*,#8586,.F.);
#11621=ORIENTED_EDGE('',*,*,#8587,.F.);
#11622=ORIENTED_EDGE('',*,*,#8588,.T.);
#11623=ORIENTED_EDGE('',*,*,#8583,.T.);
#11624=ORIENTED_EDGE('',*,*,#8575,.F.);
#11625=ORIENTED_EDGE('',*,*,#8589,.T.);
#11626=ORIENTED_EDGE('',*,*,#8590,.T.);
#11627=ORIENTED_EDGE('',*,*,#8591,.T.);
#11628=ORIENTED_EDGE('',*,*,#8592,.T.);
#11629=ORIENTED_EDGE('',*,*,#8592,.F.);
#11630=ORIENTED_EDGE('',*,*,#8593,.F.);
#11631=ORIENTED_EDGE('',*,*,#8594,.T.);
#11632=ORIENTED_EDGE('',*,*,#8595,.F.);
#11633=ORIENTED_EDGE('',*,*,#8596,.F.);
#11634=ORIENTED_EDGE('',*,*,#8597,.F.);
#11635=ORIENTED_EDGE('',*,*,#8598,.F.);
#11636=ORIENTED_EDGE('',*,*,#8599,.T.);
#11637=ORIENTED_EDGE('',*,*,#8600,.T.);
#11638=ORIENTED_EDGE('',*,*,#8601,.T.);
#11639=ORIENTED_EDGE('',*,*,#8602,.T.);
#11640=ORIENTED_EDGE('',*,*,#8603,.T.);
#11641=ORIENTED_EDGE('',*,*,#8593,.T.);
#11642=ORIENTED_EDGE('',*,*,#8591,.F.);
#11643=ORIENTED_EDGE('',*,*,#8604,.T.);
#11644=ORIENTED_EDGE('',*,*,#8602,.F.);
#11645=ORIENTED_EDGE('',*,*,#8605,.T.);
#11646=ORIENTED_EDGE('',*,*,#8601,.F.);
#11647=ORIENTED_EDGE('',*,*,#8606,.F.);
#11648=ORIENTED_EDGE('',*,*,#8607,.F.);
#11649=ORIENTED_EDGE('',*,*,#8608,.F.);
#11650=ORIENTED_EDGE('',*,*,#8609,.T.);
#11651=ORIENTED_EDGE('',*,*,#8610,.T.);
#11652=ORIENTED_EDGE('',*,*,#8605,.F.);
#11653=ORIENTED_EDGE('',*,*,#8600,.F.);
#11654=ORIENTED_EDGE('',*,*,#8611,.F.);
#11655=ORIENTED_EDGE('',*,*,#8612,.F.);
#11656=ORIENTED_EDGE('',*,*,#8613,.T.);
#11657=ORIENTED_EDGE('',*,*,#8614,.T.);
#11658=ORIENTED_EDGE('',*,*,#8606,.T.);
#11659=ORIENTED_EDGE('',*,*,#8615,.F.);
#11660=ORIENTED_EDGE('',*,*,#8616,.T.);
#11661=ORIENTED_EDGE('',*,*,#8617,.F.);
#11662=ORIENTED_EDGE('',*,*,#8618,.F.);
#11663=ORIENTED_EDGE('',*,*,#8619,.T.);
#11664=ORIENTED_EDGE('',*,*,#8620,.F.);
#11665=ORIENTED_EDGE('',*,*,#8621,.F.);
#11666=ORIENTED_EDGE('',*,*,#8622,.F.);
#11667=ORIENTED_EDGE('',*,*,#8623,.T.);
#11668=ORIENTED_EDGE('',*,*,#8624,.F.);
#11669=ORIENTED_EDGE('',*,*,#8625,.F.);
#11670=ORIENTED_EDGE('',*,*,#8626,.F.);
#11671=ORIENTED_EDGE('',*,*,#8627,.T.);
#11672=ORIENTED_EDGE('',*,*,#8628,.F.);
#11673=ORIENTED_EDGE('',*,*,#8629,.F.);
#11674=ORIENTED_EDGE('',*,*,#8630,.F.);
#11675=ORIENTED_EDGE('',*,*,#8611,.T.);
#11676=ORIENTED_EDGE('',*,*,#8599,.F.);
#11677=ORIENTED_EDGE('',*,*,#8604,.F.);
#11678=ORIENTED_EDGE('',*,*,#8590,.F.);
#11679=ORIENTED_EDGE('',*,*,#8631,.T.);
#11680=ORIENTED_EDGE('',*,*,#8570,.F.);
#11681=ORIENTED_EDGE('',*,*,#8574,.F.);
#11682=ORIENTED_EDGE('',*,*,#8568,.F.);
#11683=ORIENTED_EDGE('',*,*,#8632,.T.);
#11684=ORIENTED_EDGE('',*,*,#8547,.F.);
#11685=ORIENTED_EDGE('',*,*,#8551,.F.);
#11686=ORIENTED_EDGE('',*,*,#8545,.F.);
#11687=ORIENTED_EDGE('',*,*,#8633,.T.);
#11688=ORIENTED_EDGE('',*,*,#8524,.F.);
#11689=ORIENTED_EDGE('',*,*,#8528,.F.);
#11690=ORIENTED_EDGE('',*,*,#8522,.F.);
#11691=ORIENTED_EDGE('',*,*,#8634,.T.);
#11692=ORIENTED_EDGE('',*,*,#8501,.F.);
#11693=ORIENTED_EDGE('',*,*,#8505,.F.);
#11694=ORIENTED_EDGE('',*,*,#8499,.F.);
#11695=ORIENTED_EDGE('',*,*,#8635,.T.);
#11696=ORIENTED_EDGE('',*,*,#8636,.F.);
#11697=ORIENTED_EDGE('',*,*,#8637,.F.);
#11698=ORIENTED_EDGE('',*,*,#8638,.F.);
#11699=ORIENTED_EDGE('',*,*,#8639,.T.);
#11700=ORIENTED_EDGE('',*,*,#8640,.F.);
#11701=ORIENTED_EDGE('',*,*,#8641,.F.);
#11702=ORIENTED_EDGE('',*,*,#8642,.F.);
#11703=ORIENTED_EDGE('',*,*,#8643,.T.);
#11704=ORIENTED_EDGE('',*,*,#8644,.F.);
#11705=ORIENTED_EDGE('',*,*,#8645,.F.);
#11706=ORIENTED_EDGE('',*,*,#8646,.F.);
#11707=ORIENTED_EDGE('',*,*,#8647,.T.);
#11708=ORIENTED_EDGE('',*,*,#8648,.F.);
#11709=ORIENTED_EDGE('',*,*,#8649,.F.);
#11710=ORIENTED_EDGE('',*,*,#8650,.F.);
#11711=ORIENTED_EDGE('',*,*,#8651,.T.);
#11712=ORIENTED_EDGE('',*,*,#8652,.F.);
#11713=ORIENTED_EDGE('',*,*,#8653,.F.);
#11714=ORIENTED_EDGE('',*,*,#8616,.F.);
#11715=ORIENTED_EDGE('',*,*,#8654,.T.);
#11716=ORIENTED_EDGE('',*,*,#8612,.T.);
#11717=ORIENTED_EDGE('',*,*,#8630,.T.);
#11718=ORIENTED_EDGE('',*,*,#8655,.T.);
#11719=ORIENTED_EDGE('',*,*,#8628,.T.);
#11720=ORIENTED_EDGE('',*,*,#8656,.T.);
#11721=ORIENTED_EDGE('',*,*,#8657,.T.);
#11722=ORIENTED_EDGE('',*,*,#8658,.T.);
#11723=ORIENTED_EDGE('',*,*,#8629,.T.);
#11724=ORIENTED_EDGE('',*,*,#8658,.F.);
#11725=ORIENTED_EDGE('',*,*,#8659,.T.);
#11726=ORIENTED_EDGE('',*,*,#8660,.T.);
#11727=ORIENTED_EDGE('',*,*,#8661,.T.);
#11728=ORIENTED_EDGE('',*,*,#8655,.F.);
#11729=ORIENTED_EDGE('',*,*,#8654,.F.);
#11730=ORIENTED_EDGE('',*,*,#8661,.F.);
#11731=ORIENTED_EDGE('',*,*,#8662,.T.);
#11732=ORIENTED_EDGE('',*,*,#8663,.F.);
#11733=ORIENTED_EDGE('',*,*,#8664,.F.);
#11734=ORIENTED_EDGE('',*,*,#8665,.F.);
#11735=ORIENTED_EDGE('',*,*,#8613,.F.);
#11736=ORIENTED_EDGE('',*,*,#8660,.F.);
#11737=ORIENTED_EDGE('',*,*,#8666,.F.);
#11738=ORIENTED_EDGE('',*,*,#8667,.F.);
#11739=ORIENTED_EDGE('',*,*,#8662,.F.);
#11740=ORIENTED_EDGE('',*,*,#8657,.F.);
#11741=ORIENTED_EDGE('',*,*,#8668,.F.);
#11742=ORIENTED_EDGE('',*,*,#8669,.F.);
#11743=ORIENTED_EDGE('',*,*,#8670,.F.);
#11744=ORIENTED_EDGE('',*,*,#8671,.T.);
#11745=ORIENTED_EDGE('',*,*,#8666,.T.);
#11746=ORIENTED_EDGE('',*,*,#8659,.F.);
#11747=ORIENTED_EDGE('',*,*,#8672,.T.);
#11748=ORIENTED_EDGE('',*,*,#8673,.T.);
#11749=ORIENTED_EDGE('',*,*,#8626,.T.);
#11750=ORIENTED_EDGE('',*,*,#8674,.T.);
#11751=ORIENTED_EDGE('',*,*,#8624,.T.);
#11752=ORIENTED_EDGE('',*,*,#8675,.T.);
#11753=ORIENTED_EDGE('',*,*,#8676,.T.);
#11754=ORIENTED_EDGE('',*,*,#8677,.T.);
#11755=ORIENTED_EDGE('',*,*,#8625,.T.);
#11756=ORIENTED_EDGE('',*,*,#8677,.F.);
#11757=ORIENTED_EDGE('',*,*,#8678,.T.);
#11758=ORIENTED_EDGE('',*,*,#8679,.T.);
#11759=ORIENTED_EDGE('',*,*,#8680,.T.);
#11760=ORIENTED_EDGE('',*,*,#8674,.F.);
#11761=ORIENTED_EDGE('',*,*,#8672,.F.);
#11762=ORIENTED_EDGE('',*,*,#8680,.F.);
#11763=ORIENTED_EDGE('',*,*,#8681,.T.);
#11764=ORIENTED_EDGE('',*,*,#8682,.F.);
#11765=ORIENTED_EDGE('',*,*,#8683,.F.);
#11766=ORIENTED_EDGE('',*,*,#8684,.F.);
#11767=ORIENTED_EDGE('',*,*,#8685,.F.);
#11768=ORIENTED_EDGE('',*,*,#8679,.F.);
#11769=ORIENTED_EDGE('',*,*,#8686,.F.);
#11770=ORIENTED_EDGE('',*,*,#8687,.F.);
#11771=ORIENTED_EDGE('',*,*,#8681,.F.);
#11772=ORIENTED_EDGE('',*,*,#8676,.F.);
#11773=ORIENTED_EDGE('',*,*,#8688,.F.);
#11774=ORIENTED_EDGE('',*,*,#8689,.F.);
#11775=ORIENTED_EDGE('',*,*,#8690,.F.);
#11776=ORIENTED_EDGE('',*,*,#8691,.T.);
#11777=ORIENTED_EDGE('',*,*,#8686,.T.);
#11778=ORIENTED_EDGE('',*,*,#8678,.F.);
#11779=ORIENTED_EDGE('',*,*,#8692,.T.);
#11780=ORIENTED_EDGE('',*,*,#8693,.T.);
#11781=ORIENTED_EDGE('',*,*,#8694,.T.);
#11782=ORIENTED_EDGE('',*,*,#8695,.T.);
#11783=ORIENTED_EDGE('',*,*,#8693,.F.);
#11784=ORIENTED_EDGE('',*,*,#8696,.T.);
#11785=ORIENTED_EDGE('',*,*,#8697,.T.);
#11786=ORIENTED_EDGE('',*,*,#8698,.F.);
#11787=ORIENTED_EDGE('',*,*,#8699,.T.);
#11788=ORIENTED_EDGE('',*,*,#8700,.T.);
#11789=ORIENTED_EDGE('',*,*,#8701,.T.);
#11790=ORIENTED_EDGE('',*,*,#8702,.T.);
#11791=ORIENTED_EDGE('',*,*,#8700,.F.);
#11792=ORIENTED_EDGE('',*,*,#8703,.T.);
#11793=ORIENTED_EDGE('',*,*,#8704,.T.);
#11794=ORIENTED_EDGE('',*,*,#8705,.F.);
#11795=ORIENTED_EDGE('',*,*,#8706,.T.);
#11796=ORIENTED_EDGE('',*,*,#8707,.T.);
#11797=ORIENTED_EDGE('',*,*,#8708,.T.);
#11798=ORIENTED_EDGE('',*,*,#8709,.T.);
#11799=ORIENTED_EDGE('',*,*,#8707,.F.);
#11800=ORIENTED_EDGE('',*,*,#8710,.T.);
#11801=ORIENTED_EDGE('',*,*,#8711,.T.);
#11802=ORIENTED_EDGE('',*,*,#8712,.F.);
#11803=ORIENTED_EDGE('',*,*,#8713,.T.);
#11804=ORIENTED_EDGE('',*,*,#8714,.T.);
#11805=ORIENTED_EDGE('',*,*,#8715,.T.);
#11806=ORIENTED_EDGE('',*,*,#8716,.T.);
#11807=ORIENTED_EDGE('',*,*,#8714,.F.);
#11808=ORIENTED_EDGE('',*,*,#8717,.T.);
#11809=ORIENTED_EDGE('',*,*,#8718,.T.);
#11810=ORIENTED_EDGE('',*,*,#8719,.F.);
#11811=ORIENTED_EDGE('',*,*,#8720,.T.);
#11812=ORIENTED_EDGE('',*,*,#8721,.T.);
#11813=ORIENTED_EDGE('',*,*,#8722,.T.);
#11814=ORIENTED_EDGE('',*,*,#8723,.T.);
#11815=ORIENTED_EDGE('',*,*,#8721,.F.);
#11816=ORIENTED_EDGE('',*,*,#8724,.T.);
#11817=ORIENTED_EDGE('',*,*,#8725,.T.);
#11818=ORIENTED_EDGE('',*,*,#8726,.F.);
#11819=ORIENTED_EDGE('',*,*,#8683,.T.);
#11820=ORIENTED_EDGE('',*,*,#8727,.T.);
#11821=ORIENTED_EDGE('',*,*,#8690,.T.);
#11822=ORIENTED_EDGE('',*,*,#8728,.T.);
#11823=ORIENTED_EDGE('',*,*,#8727,.F.);
#11824=ORIENTED_EDGE('',*,*,#8682,.T.);
#11825=ORIENTED_EDGE('',*,*,#8687,.T.);
#11826=ORIENTED_EDGE('',*,*,#8691,.F.);
#11827=ORIENTED_EDGE('',*,*,#8664,.T.);
#11828=ORIENTED_EDGE('',*,*,#8729,.T.);
#11829=ORIENTED_EDGE('',*,*,#8670,.T.);
#11830=ORIENTED_EDGE('',*,*,#8730,.T.);
#11831=ORIENTED_EDGE('',*,*,#8729,.F.);
#11832=ORIENTED_EDGE('',*,*,#8663,.T.);
#11833=ORIENTED_EDGE('',*,*,#8667,.T.);
#11834=ORIENTED_EDGE('',*,*,#8671,.F.);
#11835=ORIENTED_EDGE('',*,*,#8596,.T.);
#11836=ORIENTED_EDGE('',*,*,#8731,.T.);
#11837=ORIENTED_EDGE('',*,*,#8608,.T.);
#11838=ORIENTED_EDGE('',*,*,#8732,.T.);
#11839=ORIENTED_EDGE('',*,*,#8731,.F.);
#11840=ORIENTED_EDGE('',*,*,#8595,.T.);
#11841=ORIENTED_EDGE('',*,*,#8733,.T.);
#11842=ORIENTED_EDGE('',*,*,#8609,.F.);
#11843=ORIENTED_EDGE('',*,*,#8580,.T.);
#11844=ORIENTED_EDGE('',*,*,#8734,.T.);
#11845=ORIENTED_EDGE('',*,*,#8587,.T.);
#11846=ORIENTED_EDGE('',*,*,#8735,.T.);
#11847=ORIENTED_EDGE('',*,*,#8734,.F.);
#11848=ORIENTED_EDGE('',*,*,#8579,.T.);
#11849=ORIENTED_EDGE('',*,*,#8584,.T.);
#11850=ORIENTED_EDGE('',*,*,#8588,.F.);
#11851=ORIENTED_EDGE('',*,*,#8557,.T.);
#11852=ORIENTED_EDGE('',*,*,#8736,.T.);
#11853=ORIENTED_EDGE('',*,*,#8564,.T.);
#11854=ORIENTED_EDGE('',*,*,#8737,.T.);
#11855=ORIENTED_EDGE('',*,*,#8736,.F.);
#11856=ORIENTED_EDGE('',*,*,#8556,.T.);
#11857=ORIENTED_EDGE('',*,*,#8561,.T.);
#11858=ORIENTED_EDGE('',*,*,#8565,.F.);
#11859=ORIENTED_EDGE('',*,*,#8534,.T.);
#11860=ORIENTED_EDGE('',*,*,#8738,.T.);
#11861=ORIENTED_EDGE('',*,*,#8541,.T.);
#11862=ORIENTED_EDGE('',*,*,#8739,.T.);
#11863=ORIENTED_EDGE('',*,*,#8738,.F.);
#11864=ORIENTED_EDGE('',*,*,#8533,.T.);
#11865=ORIENTED_EDGE('',*,*,#8538,.T.);
#11866=ORIENTED_EDGE('',*,*,#8542,.F.);
#11867=ORIENTED_EDGE('',*,*,#8511,.T.);
#11868=ORIENTED_EDGE('',*,*,#8740,.T.);
#11869=ORIENTED_EDGE('',*,*,#8518,.T.);
#11870=ORIENTED_EDGE('',*,*,#8741,.T.);
#11871=ORIENTED_EDGE('',*,*,#8740,.F.);
#11872=ORIENTED_EDGE('',*,*,#8510,.T.);
#11873=ORIENTED_EDGE('',*,*,#8515,.T.);
#11874=ORIENTED_EDGE('',*,*,#8519,.F.);
#11875=ORIENTED_EDGE('',*,*,#8742,.T.);
#11876=ORIENTED_EDGE('',*,*,#8743,.T.);
#11877=ORIENTED_EDGE('',*,*,#8622,.T.);
#11878=ORIENTED_EDGE('',*,*,#8744,.T.);
#11879=ORIENTED_EDGE('',*,*,#8620,.T.);
#11880=ORIENTED_EDGE('',*,*,#8745,.T.);
#11881=ORIENTED_EDGE('',*,*,#8746,.T.);
#11882=ORIENTED_EDGE('',*,*,#8747,.T.);
#11883=ORIENTED_EDGE('',*,*,#8621,.T.);
#11884=ORIENTED_EDGE('',*,*,#8747,.F.);
#11885=ORIENTED_EDGE('',*,*,#8748,.T.);
#11886=ORIENTED_EDGE('',*,*,#8749,.T.);
#11887=ORIENTED_EDGE('',*,*,#8750,.T.);
#11888=ORIENTED_EDGE('',*,*,#8744,.F.);
#11889=ORIENTED_EDGE('',*,*,#8742,.F.);
#11890=ORIENTED_EDGE('',*,*,#8750,.F.);
#11891=ORIENTED_EDGE('',*,*,#8751,.T.);
#11892=ORIENTED_EDGE('',*,*,#8724,.F.);
#11893=ORIENTED_EDGE('',*,*,#8720,.F.);
#11894=ORIENTED_EDGE('',*,*,#8752,.F.);
#11895=ORIENTED_EDGE('',*,*,#8753,.F.);
#11896=ORIENTED_EDGE('',*,*,#8749,.F.);
#11897=ORIENTED_EDGE('',*,*,#8754,.F.);
#11898=ORIENTED_EDGE('',*,*,#8725,.F.);
#11899=ORIENTED_EDGE('',*,*,#8751,.F.);
#11900=ORIENTED_EDGE('',*,*,#8746,.F.);
#11901=ORIENTED_EDGE('',*,*,#8755,.F.);
#11902=ORIENTED_EDGE('',*,*,#8756,.F.);
#11903=ORIENTED_EDGE('',*,*,#8722,.F.);
#11904=ORIENTED_EDGE('',*,*,#8726,.T.);
#11905=ORIENTED_EDGE('',*,*,#8754,.T.);
#11906=ORIENTED_EDGE('',*,*,#8748,.F.);
#11907=ORIENTED_EDGE('',*,*,#8757,.T.);
#11908=ORIENTED_EDGE('',*,*,#8758,.T.);
#11909=ORIENTED_EDGE('',*,*,#8618,.T.);
#11910=ORIENTED_EDGE('',*,*,#8759,.T.);
#11911=ORIENTED_EDGE('',*,*,#8652,.T.);
#11912=ORIENTED_EDGE('',*,*,#8760,.T.);
#11913=ORIENTED_EDGE('',*,*,#8761,.T.);
#11914=ORIENTED_EDGE('',*,*,#8762,.T.);
#11915=ORIENTED_EDGE('',*,*,#8617,.T.);
#11916=ORIENTED_EDGE('',*,*,#8653,.T.);
#11917=ORIENTED_EDGE('',*,*,#8762,.F.);
#11918=ORIENTED_EDGE('',*,*,#8763,.T.);
#11919=ORIENTED_EDGE('',*,*,#8764,.T.);
#11920=ORIENTED_EDGE('',*,*,#8765,.T.);
#11921=ORIENTED_EDGE('',*,*,#8759,.F.);
#11922=ORIENTED_EDGE('',*,*,#8757,.F.);
#11923=ORIENTED_EDGE('',*,*,#8765,.F.);
#11924=ORIENTED_EDGE('',*,*,#8766,.T.);
#11925=ORIENTED_EDGE('',*,*,#8717,.F.);
#11926=ORIENTED_EDGE('',*,*,#8713,.F.);
#11927=ORIENTED_EDGE('',*,*,#8767,.F.);
#11928=ORIENTED_EDGE('',*,*,#8768,.F.);
#11929=ORIENTED_EDGE('',*,*,#8764,.F.);
#11930=ORIENTED_EDGE('',*,*,#8769,.F.);
#11931=ORIENTED_EDGE('',*,*,#8718,.F.);
#11932=ORIENTED_EDGE('',*,*,#8766,.F.);
#11933=ORIENTED_EDGE('',*,*,#8761,.F.);
#11934=ORIENTED_EDGE('',*,*,#8770,.F.);
#11935=ORIENTED_EDGE('',*,*,#8771,.F.);
#11936=ORIENTED_EDGE('',*,*,#8715,.F.);
#11937=ORIENTED_EDGE('',*,*,#8719,.T.);
#11938=ORIENTED_EDGE('',*,*,#8769,.T.);
#11939=ORIENTED_EDGE('',*,*,#8763,.F.);
#11940=ORIENTED_EDGE('',*,*,#8772,.T.);
#11941=ORIENTED_EDGE('',*,*,#8773,.T.);
#11942=ORIENTED_EDGE('',*,*,#8650,.T.);
#11943=ORIENTED_EDGE('',*,*,#8774,.T.);
#11944=ORIENTED_EDGE('',*,*,#8648,.T.);
#11945=ORIENTED_EDGE('',*,*,#8775,.T.);
#11946=ORIENTED_EDGE('',*,*,#8776,.T.);
#11947=ORIENTED_EDGE('',*,*,#8777,.T.);
#11948=ORIENTED_EDGE('',*,*,#8649,.T.);
#11949=ORIENTED_EDGE('',*,*,#8777,.F.);
#11950=ORIENTED_EDGE('',*,*,#8778,.T.);
#11951=ORIENTED_EDGE('',*,*,#8779,.T.);
#11952=ORIENTED_EDGE('',*,*,#8780,.T.);
#11953=ORIENTED_EDGE('',*,*,#8774,.F.);
#11954=ORIENTED_EDGE('',*,*,#8772,.F.);
#11955=ORIENTED_EDGE('',*,*,#8780,.F.);
#11956=ORIENTED_EDGE('',*,*,#8781,.T.);
#11957=ORIENTED_EDGE('',*,*,#8710,.F.);
#11958=ORIENTED_EDGE('',*,*,#8706,.F.);
#11959=ORIENTED_EDGE('',*,*,#8782,.F.);
#11960=ORIENTED_EDGE('',*,*,#8783,.F.);
#11961=ORIENTED_EDGE('',*,*,#8779,.F.);
#11962=ORIENTED_EDGE('',*,*,#8784,.F.);
#11963=ORIENTED_EDGE('',*,*,#8711,.F.);
#11964=ORIENTED_EDGE('',*,*,#8781,.F.);
#11965=ORIENTED_EDGE('',*,*,#8776,.F.);
#11966=ORIENTED_EDGE('',*,*,#8785,.F.);
#11967=ORIENTED_EDGE('',*,*,#8786,.F.);
#11968=ORIENTED_EDGE('',*,*,#8708,.F.);
#11969=ORIENTED_EDGE('',*,*,#8712,.T.);
#11970=ORIENTED_EDGE('',*,*,#8784,.T.);
#11971=ORIENTED_EDGE('',*,*,#8778,.F.);
#11972=ORIENTED_EDGE('',*,*,#8787,.T.);
#11973=ORIENTED_EDGE('',*,*,#8788,.T.);
#11974=ORIENTED_EDGE('',*,*,#8646,.T.);
#11975=ORIENTED_EDGE('',*,*,#8789,.T.);
#11976=ORIENTED_EDGE('',*,*,#8644,.T.);
#11977=ORIENTED_EDGE('',*,*,#8790,.T.);
#11978=ORIENTED_EDGE('',*,*,#8791,.T.);
#11979=ORIENTED_EDGE('',*,*,#8792,.T.);
#11980=ORIENTED_EDGE('',*,*,#8645,.T.);
#11981=ORIENTED_EDGE('',*,*,#8792,.F.);
#11982=ORIENTED_EDGE('',*,*,#8793,.T.);
#11983=ORIENTED_EDGE('',*,*,#8794,.T.);
#11984=ORIENTED_EDGE('',*,*,#8795,.T.);
#11985=ORIENTED_EDGE('',*,*,#8789,.F.);
#11986=ORIENTED_EDGE('',*,*,#8787,.F.);
#11987=ORIENTED_EDGE('',*,*,#8795,.F.);
#11988=ORIENTED_EDGE('',*,*,#8796,.T.);
#11989=ORIENTED_EDGE('',*,*,#8703,.F.);
#11990=ORIENTED_EDGE('',*,*,#8699,.F.);
#11991=ORIENTED_EDGE('',*,*,#8797,.F.);
#11992=ORIENTED_EDGE('',*,*,#8798,.F.);
#11993=ORIENTED_EDGE('',*,*,#8794,.F.);
#11994=ORIENTED_EDGE('',*,*,#8799,.F.);
#11995=ORIENTED_EDGE('',*,*,#8704,.F.);
#11996=ORIENTED_EDGE('',*,*,#8796,.F.);
#11997=ORIENTED_EDGE('',*,*,#8791,.F.);
#11998=ORIENTED_EDGE('',*,*,#8800,.F.);
#11999=ORIENTED_EDGE('',*,*,#8801,.F.);
#12000=ORIENTED_EDGE('',*,*,#8701,.F.);
#12001=ORIENTED_EDGE('',*,*,#8705,.T.);
#12002=ORIENTED_EDGE('',*,*,#8799,.T.);
#12003=ORIENTED_EDGE('',*,*,#8793,.F.);
#12004=ORIENTED_EDGE('',*,*,#8802,.T.);
#12005=ORIENTED_EDGE('',*,*,#8803,.T.);
#12006=ORIENTED_EDGE('',*,*,#8642,.T.);
#12007=ORIENTED_EDGE('',*,*,#8804,.T.);
#12008=ORIENTED_EDGE('',*,*,#8640,.T.);
#12009=ORIENTED_EDGE('',*,*,#8805,.T.);
#12010=ORIENTED_EDGE('',*,*,#8806,.T.);
#12011=ORIENTED_EDGE('',*,*,#8807,.T.);
#12012=ORIENTED_EDGE('',*,*,#8641,.T.);
#12013=ORIENTED_EDGE('',*,*,#8807,.F.);
#12014=ORIENTED_EDGE('',*,*,#8808,.T.);
#12015=ORIENTED_EDGE('',*,*,#8809,.T.);
#12016=ORIENTED_EDGE('',*,*,#8810,.T.);
#12017=ORIENTED_EDGE('',*,*,#8804,.F.);
#12018=ORIENTED_EDGE('',*,*,#8809,.F.);
#12019=ORIENTED_EDGE('',*,*,#8811,.F.);
#12020=ORIENTED_EDGE('',*,*,#8697,.F.);
#12021=ORIENTED_EDGE('',*,*,#8812,.F.);
#12022=ORIENTED_EDGE('',*,*,#8806,.F.);
#12023=ORIENTED_EDGE('',*,*,#8813,.F.);
#12024=ORIENTED_EDGE('',*,*,#8814,.F.);
#12025=ORIENTED_EDGE('',*,*,#8694,.F.);
#12026=ORIENTED_EDGE('',*,*,#8698,.T.);
#12027=ORIENTED_EDGE('',*,*,#8811,.T.);
#12028=ORIENTED_EDGE('',*,*,#8808,.F.);
#12029=ORIENTED_EDGE('',*,*,#8805,.F.);
#12030=ORIENTED_EDGE('',*,*,#8639,.F.);
#12031=ORIENTED_EDGE('',*,*,#8815,.F.);
#12032=ORIENTED_EDGE('',*,*,#8816,.T.);
#12033=ORIENTED_EDGE('',*,*,#8817,.T.);
#12034=ORIENTED_EDGE('',*,*,#8813,.T.);
#12035=ORIENTED_EDGE('',*,*,#8818,.T.);
#12036=ORIENTED_EDGE('',*,*,#8819,.T.);
#12037=ORIENTED_EDGE('',*,*,#8820,.T.);
#12038=ORIENTED_EDGE('',*,*,#8821,.T.);
#12039=ORIENTED_EDGE('',*,*,#8819,.F.);
#12040=ORIENTED_EDGE('',*,*,#8822,.T.);
#12041=ORIENTED_EDGE('',*,*,#8823,.T.);
#12042=ORIENTED_EDGE('',*,*,#8824,.F.);
#12043=ORIENTED_EDGE('',*,*,#8825,.T.);
#12044=ORIENTED_EDGE('',*,*,#8815,.T.);
#12045=ORIENTED_EDGE('',*,*,#8638,.T.);
#12046=ORIENTED_EDGE('',*,*,#8826,.T.);
#12047=ORIENTED_EDGE('',*,*,#8636,.T.);
#12048=ORIENTED_EDGE('',*,*,#8827,.T.);
#12049=ORIENTED_EDGE('',*,*,#8828,.T.);
#12050=ORIENTED_EDGE('',*,*,#8829,.T.);
#12051=ORIENTED_EDGE('',*,*,#8637,.T.);
#12052=ORIENTED_EDGE('',*,*,#8829,.F.);
#12053=ORIENTED_EDGE('',*,*,#8830,.T.);
#12054=ORIENTED_EDGE('',*,*,#8831,.T.);
#12055=ORIENTED_EDGE('',*,*,#8832,.T.);
#12056=ORIENTED_EDGE('',*,*,#8826,.F.);
#12057=ORIENTED_EDGE('',*,*,#8831,.F.);
#12058=ORIENTED_EDGE('',*,*,#8833,.F.);
#12059=ORIENTED_EDGE('',*,*,#8823,.F.);
#12060=ORIENTED_EDGE('',*,*,#8834,.F.);
#12061=ORIENTED_EDGE('',*,*,#8828,.F.);
#12062=ORIENTED_EDGE('',*,*,#8835,.F.);
#12063=ORIENTED_EDGE('',*,*,#8836,.F.);
#12064=ORIENTED_EDGE('',*,*,#8820,.F.);
#12065=ORIENTED_EDGE('',*,*,#8824,.T.);
#12066=ORIENTED_EDGE('',*,*,#8833,.T.);
#12067=ORIENTED_EDGE('',*,*,#8830,.F.);
#12068=ORIENTED_EDGE('',*,*,#8498,.F.);
#12069=ORIENTED_EDGE('',*,*,#8513,.T.);
#12070=ORIENTED_EDGE('',*,*,#8837,.T.);
#12071=ORIENTED_EDGE('',*,*,#8835,.T.);
#12072=ORIENTED_EDGE('',*,*,#8827,.F.);
#12073=ORIENTED_EDGE('',*,*,#8635,.F.);
#12074=ORIENTED_EDGE('',*,*,#8838,.T.);
#12075=ORIENTED_EDGE('',*,*,#8839,.T.);
#12076=ORIENTED_EDGE('',*,*,#8840,.T.);
#12077=ORIENTED_EDGE('',*,*,#8839,.F.);
#12078=ORIENTED_EDGE('',*,*,#8840,.F.);
#12079=ORIENTED_EDGE('',*,*,#8841,.T.);
#12080=ORIENTED_EDGE('',*,*,#8842,.T.);
#12081=ORIENTED_EDGE('',*,*,#8841,.F.);
#12082=ORIENTED_EDGE('',*,*,#8814,.T.);
#12083=ORIENTED_EDGE('',*,*,#8817,.F.);
#12084=ORIENTED_EDGE('',*,*,#8843,.T.);
#12085=ORIENTED_EDGE('',*,*,#8821,.F.);
#12086=ORIENTED_EDGE('',*,*,#8836,.T.);
#12087=ORIENTED_EDGE('',*,*,#8837,.F.);
#12088=ORIENTED_EDGE('',*,*,#8512,.T.);
#12089=ORIENTED_EDGE('',*,*,#8741,.F.);
#12090=ORIENTED_EDGE('',*,*,#8517,.T.);
#12091=ORIENTED_EDGE('',*,*,#8844,.F.);
#12092=ORIENTED_EDGE('',*,*,#8535,.T.);
#12093=ORIENTED_EDGE('',*,*,#8739,.F.);
#12094=ORIENTED_EDGE('',*,*,#8540,.T.);
#12095=ORIENTED_EDGE('',*,*,#8845,.F.);
#12096=ORIENTED_EDGE('',*,*,#8558,.T.);
#12097=ORIENTED_EDGE('',*,*,#8737,.F.);
#12098=ORIENTED_EDGE('',*,*,#8563,.T.);
#12099=ORIENTED_EDGE('',*,*,#8846,.F.);
#12100=ORIENTED_EDGE('',*,*,#8581,.T.);
#12101=ORIENTED_EDGE('',*,*,#8735,.F.);
#12102=ORIENTED_EDGE('',*,*,#8586,.T.);
#12103=ORIENTED_EDGE('',*,*,#8847,.F.);
#12104=ORIENTED_EDGE('',*,*,#8597,.T.);
#12105=ORIENTED_EDGE('',*,*,#8732,.F.);
#12106=ORIENTED_EDGE('',*,*,#8607,.T.);
#12107=ORIENTED_EDGE('',*,*,#8614,.F.);
#12108=ORIENTED_EDGE('',*,*,#8665,.T.);
#12109=ORIENTED_EDGE('',*,*,#8730,.F.);
#12110=ORIENTED_EDGE('',*,*,#8669,.T.);
#12111=ORIENTED_EDGE('',*,*,#8848,.F.);
#12112=ORIENTED_EDGE('',*,*,#8684,.T.);
#12113=ORIENTED_EDGE('',*,*,#8728,.F.);
#12114=ORIENTED_EDGE('',*,*,#8689,.T.);
#12115=ORIENTED_EDGE('',*,*,#8849,.F.);
#12116=ORIENTED_EDGE('',*,*,#8752,.T.);
#12117=ORIENTED_EDGE('',*,*,#8723,.F.);
#12118=ORIENTED_EDGE('',*,*,#8756,.T.);
#12119=ORIENTED_EDGE('',*,*,#8850,.F.);
#12120=ORIENTED_EDGE('',*,*,#8767,.T.);
#12121=ORIENTED_EDGE('',*,*,#8716,.F.);
#12122=ORIENTED_EDGE('',*,*,#8771,.T.);
#12123=ORIENTED_EDGE('',*,*,#8851,.F.);
#12124=ORIENTED_EDGE('',*,*,#8782,.T.);
#12125=ORIENTED_EDGE('',*,*,#8709,.F.);
#12126=ORIENTED_EDGE('',*,*,#8786,.T.);
#12127=ORIENTED_EDGE('',*,*,#8852,.F.);
#12128=ORIENTED_EDGE('',*,*,#8797,.T.);
#12129=ORIENTED_EDGE('',*,*,#8702,.F.);
#12130=ORIENTED_EDGE('',*,*,#8801,.T.);
#12131=ORIENTED_EDGE('',*,*,#8853,.F.);
#12132=ORIENTED_EDGE('',*,*,#8854,.T.);
#12133=ORIENTED_EDGE('',*,*,#8695,.F.);
#12134=ORIENTED_EDGE('',*,*,#8838,.F.);
#12135=ORIENTED_EDGE('',*,*,#8842,.F.);
#12136=ORIENTED_EDGE('',*,*,#8855,.F.);
#12137=ORIENTED_EDGE('',*,*,#8856,.T.);
#12138=ORIENTED_EDGE('',*,*,#8857,.T.);
#12139=ORIENTED_EDGE('',*,*,#8858,.F.);
#12140=ORIENTED_EDGE('',*,*,#8859,.F.);
#12141=ORIENTED_EDGE('',*,*,#8858,.T.);
#12142=ORIENTED_EDGE('',*,*,#8860,.T.);
#12143=ORIENTED_EDGE('',*,*,#8861,.F.);
#12144=ORIENTED_EDGE('',*,*,#8862,.F.);
#12145=ORIENTED_EDGE('',*,*,#8863,.T.);
#12146=ORIENTED_EDGE('',*,*,#8864,.T.);
#12147=ORIENTED_EDGE('',*,*,#8856,.F.);
#12148=ORIENTED_EDGE('',*,*,#8865,.F.);
#12149=ORIENTED_EDGE('',*,*,#8861,.T.);
#12150=ORIENTED_EDGE('',*,*,#8866,.T.);
#12151=ORIENTED_EDGE('',*,*,#8863,.F.);
#12152=ORIENTED_EDGE('',*,*,#8857,.F.);
#12153=ORIENTED_EDGE('',*,*,#8864,.F.);
#12154=ORIENTED_EDGE('',*,*,#8866,.F.);
#12155=ORIENTED_EDGE('',*,*,#8860,.F.);
#12156=ORIENTED_EDGE('',*,*,#8825,.F.);
#12157=ORIENTED_EDGE('',*,*,#8832,.F.);
#12158=ORIENTED_EDGE('',*,*,#8834,.T.);
#12159=ORIENTED_EDGE('',*,*,#8822,.F.);
#12160=ORIENTED_EDGE('',*,*,#8818,.F.);
#12161=ORIENTED_EDGE('',*,*,#8843,.F.);
#12162=ORIENTED_EDGE('',*,*,#8816,.F.);
#12163=ORIENTED_EDGE('',*,*,#8502,.F.);
#12164=ORIENTED_EDGE('',*,*,#8634,.F.);
#12165=ORIENTED_EDGE('',*,*,#8521,.F.);
#12166=ORIENTED_EDGE('',*,*,#8536,.T.);
#12167=ORIENTED_EDGE('',*,*,#8844,.T.);
#12168=ORIENTED_EDGE('',*,*,#8516,.T.);
#12169=ORIENTED_EDGE('',*,*,#8525,.F.);
#12170=ORIENTED_EDGE('',*,*,#8633,.F.);
#12171=ORIENTED_EDGE('',*,*,#8544,.F.);
#12172=ORIENTED_EDGE('',*,*,#8559,.T.);
#12173=ORIENTED_EDGE('',*,*,#8845,.T.);
#12174=ORIENTED_EDGE('',*,*,#8539,.T.);
#12175=ORIENTED_EDGE('',*,*,#8548,.F.);
#12176=ORIENTED_EDGE('',*,*,#8632,.F.);
#12177=ORIENTED_EDGE('',*,*,#8567,.F.);
#12178=ORIENTED_EDGE('',*,*,#8582,.T.);
#12179=ORIENTED_EDGE('',*,*,#8846,.T.);
#12180=ORIENTED_EDGE('',*,*,#8562,.T.);
#12181=ORIENTED_EDGE('',*,*,#8571,.F.);
#12182=ORIENTED_EDGE('',*,*,#8631,.F.);
#12183=ORIENTED_EDGE('',*,*,#8589,.F.);
#12184=ORIENTED_EDGE('',*,*,#8598,.T.);
#12185=ORIENTED_EDGE('',*,*,#8847,.T.);
#12186=ORIENTED_EDGE('',*,*,#8585,.T.);
#12187=ORIENTED_EDGE('',*,*,#8603,.F.);
#12188=ORIENTED_EDGE('',*,*,#8610,.F.);
#12189=ORIENTED_EDGE('',*,*,#8733,.F.);
#12190=ORIENTED_EDGE('',*,*,#8594,.F.);
#12191=ORIENTED_EDGE('',*,*,#8656,.F.);
#12192=ORIENTED_EDGE('',*,*,#8627,.F.);
#12193=ORIENTED_EDGE('',*,*,#8673,.F.);
#12194=ORIENTED_EDGE('',*,*,#8685,.T.);
#12195=ORIENTED_EDGE('',*,*,#8848,.T.);
#12196=ORIENTED_EDGE('',*,*,#8668,.T.);
#12197=ORIENTED_EDGE('',*,*,#8675,.F.);
#12198=ORIENTED_EDGE('',*,*,#8623,.F.);
#12199=ORIENTED_EDGE('',*,*,#8743,.F.);
#12200=ORIENTED_EDGE('',*,*,#8753,.T.);
#12201=ORIENTED_EDGE('',*,*,#8849,.T.);
#12202=ORIENTED_EDGE('',*,*,#8688,.T.);
#12203=ORIENTED_EDGE('',*,*,#8745,.F.);
#12204=ORIENTED_EDGE('',*,*,#8619,.F.);
#12205=ORIENTED_EDGE('',*,*,#8758,.F.);
#12206=ORIENTED_EDGE('',*,*,#8768,.T.);
#12207=ORIENTED_EDGE('',*,*,#8850,.T.);
#12208=ORIENTED_EDGE('',*,*,#8755,.T.);
#12209=ORIENTED_EDGE('',*,*,#8760,.F.);
#12210=ORIENTED_EDGE('',*,*,#8651,.F.);
#12211=ORIENTED_EDGE('',*,*,#8773,.F.);
#12212=ORIENTED_EDGE('',*,*,#8783,.T.);
#12213=ORIENTED_EDGE('',*,*,#8851,.T.);
#12214=ORIENTED_EDGE('',*,*,#8770,.T.);
#12215=ORIENTED_EDGE('',*,*,#8775,.F.);
#12216=ORIENTED_EDGE('',*,*,#8647,.F.);
#12217=ORIENTED_EDGE('',*,*,#8788,.F.);
#12218=ORIENTED_EDGE('',*,*,#8798,.T.);
#12219=ORIENTED_EDGE('',*,*,#8852,.T.);
#12220=ORIENTED_EDGE('',*,*,#8785,.T.);
#12221=ORIENTED_EDGE('',*,*,#8802,.F.);
#12222=ORIENTED_EDGE('',*,*,#8810,.F.);
#12223=ORIENTED_EDGE('',*,*,#8812,.T.);
#12224=ORIENTED_EDGE('',*,*,#8696,.F.);
#12225=ORIENTED_EDGE('',*,*,#8692,.F.);
#12226=ORIENTED_EDGE('',*,*,#8854,.F.);
#12227=ORIENTED_EDGE('',*,*,#8867,.F.);
#12228=ORIENTED_EDGE('',*,*,#8790,.F.);
#12229=ORIENTED_EDGE('',*,*,#8643,.F.);
#12230=ORIENTED_EDGE('',*,*,#8803,.F.);
#12231=ORIENTED_EDGE('',*,*,#8867,.T.);
#12232=ORIENTED_EDGE('',*,*,#8853,.T.);
#12233=ORIENTED_EDGE('',*,*,#8800,.T.);
#12234=ORIENTED_EDGE('',*,*,#8868,.F.);
#12235=ORIENTED_EDGE('',*,*,#8615,.T.);
#12236=ORIENTED_EDGE('',*,*,#8869,.F.);
#12237=ORIENTED_EDGE('',*,*,#8870,.T.);
#12238=ORIENTED_EDGE('',*,*,#8868,.T.);
#12239=ORIENTED_EDGE('',*,*,#8870,.F.);
#12240=ORIENTED_EDGE('',*,*,#8869,.T.);
#12241=ORIENTED_EDGE('',*,*,#8871,.F.);
#12242=ORIENTED_EDGE('',*,*,#8872,.F.);
#12243=ORIENTED_EDGE('',*,*,#8873,.T.);
#12244=ORIENTED_EDGE('',*,*,#8871,.T.);
#12245=ORIENTED_EDGE('',*,*,#8873,.F.);
#12246=ORIENTED_EDGE('',*,*,#8872,.T.);
#12247=ORIENTED_EDGE('',*,*,#8874,.F.);
#12248=ORIENTED_EDGE('',*,*,#8875,.F.);
#12249=ORIENTED_EDGE('',*,*,#8876,.T.);
#12250=ORIENTED_EDGE('',*,*,#8874,.T.);
#12251=ORIENTED_EDGE('',*,*,#8876,.F.);
#12252=ORIENTED_EDGE('',*,*,#8865,.T.);
#12253=ORIENTED_EDGE('',*,*,#8862,.T.);
#12254=ORIENTED_EDGE('',*,*,#8855,.T.);
#12255=ORIENTED_EDGE('',*,*,#8859,.T.);
#12256=ORIENTED_EDGE('',*,*,#8877,.F.);
#12257=ORIENTED_EDGE('',*,*,#8878,.T.);
#12258=ORIENTED_EDGE('',*,*,#8875,.T.);
#12259=ORIENTED_EDGE('',*,*,#8878,.F.);
#12260=ORIENTED_EDGE('',*,*,#8877,.T.);
#14135=CONICAL_SURFACE('',#15953,10.85,0.785398163397446);
#14136=CONICAL_SURFACE('',#15961,10.85,0.785398163397448);
#14137=CONICAL_SURFACE('',#15969,10.85,0.785398163397448);
#14138=CONICAL_SURFACE('',#15977,10.85,0.785398163397448);
#14139=CONICAL_SURFACE('',#15986,10.85,0.785398163397448);
#14140=CONICAL_SURFACE('',#15990,10.85,0.463647609000803);
#14141=CONICAL_SURFACE('',#16018,10.85,0.785398163397448);
#14142=CONICAL_SURFACE('',#16025,10.85,0.785398163397448);
#14143=CONICAL_SURFACE('',#16056,10.85,0.785398163397446);
#14144=CONICAL_SURFACE('',#16063,10.85,0.785398163397448);
#14145=CONICAL_SURFACE('',#16070,10.85,0.785398163397448);
#14146=CONICAL_SURFACE('',#16077,10.85,0.785398163397448);
#14147=CONICAL_SURFACE('',#16084,10.85,0.785398163397448);
#14148=CONICAL_SURFACE('',#16088,10.85,0.463647609000803);
#14149=CONICAL_SURFACE('',#16094,10.85,0.785398163397446);
#14150=CONICAL_SURFACE('',#16098,10.85,0.463647609000803);
#14151=CONICAL_SURFACE('',#16100,3.6,0.78539816339745);
#14152=CONICAL_SURFACE('',#16125,10.85,0.463647609000803);
#14153=CONICAL_SURFACE('',#16126,10.85,0.463647609000803);
#14154=CONICAL_SURFACE('',#16127,10.85,0.463647609000803);
#14155=CONICAL_SURFACE('',#16128,10.85,0.463647609000803);
#14156=CONICAL_SURFACE('',#16130,10.85,0.463647609000803);
#14157=CONICAL_SURFACE('',#16131,10.85,0.463647609000803);
#14158=CONICAL_SURFACE('',#16132,10.85,0.463647609000803);
#14159=CONICAL_SURFACE('',#16133,10.85,0.463647609000803);
#14160=CONICAL_SURFACE('',#16134,10.85,0.463647609000803);
#14161=CONICAL_SURFACE('',#16136,10.85,0.463647609000803);
#14162=CONICAL_SURFACE('',#16149,12.25,0.785398163397442);
#14545=ADVANCED_FACE('',(#1978),#666,.T.);
#14546=ADVANCED_FACE('',(#1979),#667,.T.);
#14547=ADVANCED_FACE('',(#1980),#14135,.T.);
#14548=ADVANCED_FACE('',(#1981),#668,.F.);
#14549=ADVANCED_FACE('',(#1982),#669,.F.);
#14550=ADVANCED_FACE('',(#1983),#670,.F.);
#14551=ADVANCED_FACE('',(#1984),#671,.T.);
#14552=ADVANCED_FACE('',(#1985),#672,.T.);
#14553=ADVANCED_FACE('',(#1986),#14136,.T.);
#14554=ADVANCED_FACE('',(#1987),#673,.F.);
#14555=ADVANCED_FACE('',(#1988),#674,.F.);
#14556=ADVANCED_FACE('',(#1989),#675,.F.);
#14557=ADVANCED_FACE('',(#1990),#676,.T.);
#14558=ADVANCED_FACE('',(#1991),#677,.T.);
#14559=ADVANCED_FACE('',(#1992),#14137,.T.);
#14560=ADVANCED_FACE('',(#1993),#678,.F.);
#14561=ADVANCED_FACE('',(#1994),#679,.F.);
#14562=ADVANCED_FACE('',(#1995),#680,.F.);
#14563=ADVANCED_FACE('',(#1996),#681,.T.);
#14564=ADVANCED_FACE('',(#1997),#682,.T.);
#14565=ADVANCED_FACE('',(#1998),#14138,.T.);
#14566=ADVANCED_FACE('',(#1999),#683,.F.);
#14567=ADVANCED_FACE('',(#2000),#684,.F.);
#14568=ADVANCED_FACE('',(#2001),#685,.F.);
#14569=ADVANCED_FACE('',(#2002),#686,.T.);
#14570=ADVANCED_FACE('',(#2003),#687,.F.);
#14571=ADVANCED_FACE('',(#2004),#688,.T.);
#14572=ADVANCED_FACE('',(#2005),#14139,.T.);
#14573=ADVANCED_FACE('',(#2006),#689,.F.);
#14574=ADVANCED_FACE('',(#2007),#14140,.T.);
#14575=ADVANCED_FACE('',(#2008),#1489,.T.);
#14576=ADVANCED_FACE('',(#2009),#690,.T.);
#14577=ADVANCED_FACE('',(#2010),#691,.T.);
#14578=ADVANCED_FACE('',(#2011),#14141,.T.);
#14579=ADVANCED_FACE('',(#2012),#692,.F.);
#14580=ADVANCED_FACE('',(#2013),#693,.F.);
#14581=ADVANCED_FACE('',(#2014),#694,.F.);
#14582=ADVANCED_FACE('',(#2015),#695,.T.);
#14583=ADVANCED_FACE('',(#2016),#696,.T.);
#14584=ADVANCED_FACE('',(#2017),#14142,.T.);
#14585=ADVANCED_FACE('',(#2018),#697,.F.);
#14586=ADVANCED_FACE('',(#2019),#698,.F.);
#14587=ADVANCED_FACE('',(#2020),#699,.F.);
#14588=ADVANCED_FACE('',(#2021),#700,.T.);
#14589=ADVANCED_FACE('',(#2022),#701,.F.);
#14590=ADVANCED_FACE('',(#2023),#702,.T.);
#14591=ADVANCED_FACE('',(#2024),#703,.F.);
#14592=ADVANCED_FACE('',(#2025),#704,.T.);
#14593=ADVANCED_FACE('',(#2026),#705,.F.);
#14594=ADVANCED_FACE('',(#2027),#706,.T.);
#14595=ADVANCED_FACE('',(#2028),#707,.F.);
#14596=ADVANCED_FACE('',(#2029),#708,.T.);
#14597=ADVANCED_FACE('',(#2030),#709,.F.);
#14598=ADVANCED_FACE('',(#2031),#710,.T.);
#14599=ADVANCED_FACE('',(#2032),#711,.F.);
#14600=ADVANCED_FACE('',(#2033),#712,.T.);
#14601=ADVANCED_FACE('',(#2034),#713,.F.);
#14602=ADVANCED_FACE('',(#2035),#714,.T.);
#14603=ADVANCED_FACE('',(#2036),#715,.F.);
#14604=ADVANCED_FACE('',(#2037),#716,.T.);
#14605=ADVANCED_FACE('',(#2038),#717,.F.);
#14606=ADVANCED_FACE('',(#2039),#718,.T.);
#14607=ADVANCED_FACE('',(#2040),#719,.F.);
#14608=ADVANCED_FACE('',(#2041),#720,.T.);
#14609=ADVANCED_FACE('',(#2042),#721,.F.);
#14610=ADVANCED_FACE('',(#2043),#722,.T.);
#14611=ADVANCED_FACE('',(#2044),#723,.F.);
#14612=ADVANCED_FACE('',(#2045),#724,.T.);
#14613=ADVANCED_FACE('',(#2046),#725,.T.);
#14614=ADVANCED_FACE('',(#2047),#14143,.T.);
#14615=ADVANCED_FACE('',(#2048),#726,.F.);
#14616=ADVANCED_FACE('',(#2049),#727,.F.);
#14617=ADVANCED_FACE('',(#2050),#728,.F.);
#14618=ADVANCED_FACE('',(#2051),#729,.T.);
#14619=ADVANCED_FACE('',(#2052),#730,.T.);
#14620=ADVANCED_FACE('',(#2053),#14144,.T.);
#14621=ADVANCED_FACE('',(#2054),#731,.F.);
#14622=ADVANCED_FACE('',(#2055),#732,.F.);
#14623=ADVANCED_FACE('',(#2056),#733,.F.);
#14624=ADVANCED_FACE('',(#2057),#734,.T.);
#14625=ADVANCED_FACE('',(#2058),#735,.T.);
#14626=ADVANCED_FACE('',(#2059),#14145,.T.);
#14627=ADVANCED_FACE('',(#2060),#736,.F.);
#14628=ADVANCED_FACE('',(#2061),#737,.F.);
#14629=ADVANCED_FACE('',(#2062),#738,.F.);
#14630=ADVANCED_FACE('',(#2063),#739,.T.);
#14631=ADVANCED_FACE('',(#2064),#740,.T.);
#14632=ADVANCED_FACE('',(#2065),#14146,.T.);
#14633=ADVANCED_FACE('',(#2066),#741,.F.);
#14634=ADVANCED_FACE('',(#2067),#742,.F.);
#14635=ADVANCED_FACE('',(#2068),#743,.F.);
#14636=ADVANCED_FACE('',(#2069),#744,.T.);
#14637=ADVANCED_FACE('',(#2070),#745,.T.);
#14638=ADVANCED_FACE('',(#2071),#14147,.T.);
#14639=ADVANCED_FACE('',(#2072),#746,.F.);
#14640=ADVANCED_FACE('',(#2073),#747,.F.);
#14641=ADVANCED_FACE('',(#2074),#14148,.T.);
#14642=ADVANCED_FACE('',(#2075),#748,.T.);
#14643=ADVANCED_FACE('',(#2076),#749,.F.);
#14644=ADVANCED_FACE('',(#2077),#750,.T.);
#14645=ADVANCED_FACE('',(#2078),#751,.T.);
#14646=ADVANCED_FACE('',(#2079),#14149,.T.);
#14647=ADVANCED_FACE('',(#2080),#752,.F.);
#14648=ADVANCED_FACE('',(#2081),#753,.F.);
#14649=ADVANCED_FACE('',(#2082),#14150,.T.);
#14650=ADVANCED_FACE('',(#2083),#14151,.F.);
#14651=ADVANCED_FACE('',(#2084),#1490,.F.);
#14652=ADVANCED_FACE('',(#2085,#486),#754,.T.);
#14653=ADVANCED_FACE('',(#2086),#755,.F.);
#14654=ADVANCED_FACE('',(#2087),#756,.F.);
#14655=ADVANCED_FACE('',(#2088),#757,.F.);
#14656=ADVANCED_FACE('',(#2089),#758,.F.);
#14657=ADVANCED_FACE('',(#2090),#759,.F.);
#14658=ADVANCED_FACE('',(#2091),#760,.F.);
#14659=ADVANCED_FACE('',(#2092),#761,.F.);
#14660=ADVANCED_FACE('',(#2093),#14152,.T.);
#14661=ADVANCED_FACE('',(#2094),#14153,.T.);
#14662=ADVANCED_FACE('',(#2095),#14154,.T.);
#14663=ADVANCED_FACE('',(#2096),#14155,.T.);
#14664=ADVANCED_FACE('',(#2097),#762,.F.);
#14665=ADVANCED_FACE('',(#2098),#14156,.T.);
#14666=ADVANCED_FACE('',(#2099),#14157,.T.);
#14667=ADVANCED_FACE('',(#2100),#14158,.T.);
#14668=ADVANCED_FACE('',(#2101),#14159,.T.);
#14669=ADVANCED_FACE('',(#2102),#14160,.T.);
#14670=ADVANCED_FACE('',(#2103),#763,.F.);
#14671=ADVANCED_FACE('',(#2104),#14161,.T.);
#14672=ADVANCED_FACE('',(#2105,#487),#764,.T.);
#14673=ADVANCED_FACE('',(#2106),#1491,.T.);
#14674=ADVANCED_FACE('',(#2107,#488),#765,.T.);
#14675=ADVANCED_FACE('',(#2108),#1492,.T.);
#14676=ADVANCED_FACE('',(#2109,#489),#766,.T.);
#14677=ADVANCED_FACE('',(#2110,#490),#1493,.T.);
#14678=ADVANCED_FACE('',(#2111),#14162,.T.);
#14679=ADVANCED_FACE('',(#2112),#767,.T.);
#15076=CLOSED_SHELL('',(#14545,#14546,#14547,#14548,#14549,#14550,#14551,
#14552,#14553,#14554,#14555,#14556,#14557,#14558,#14559,#14560,#14561,#14562,
#14563,#14564,#14565,#14566,#14567,#14568,#14569,#14570,#14571,#14572,#14573,
#14574,#14575,#14576,#14577,#14578,#14579,#14580,#14581,#14582,#14583,#14584,
#14585,#14586,#14587,#14588,#14589,#14590,#14591,#14592,#14593,#14594,#14595,
#14596,#14597,#14598,#14599,#14600,#14601,#14602,#14603,#14604,#14605,#14606,
#14607,#14608,#14609,#14610,#14611,#14612,#14613,#14614,#14615,#14616,#14617,
#14618,#14619,#14620,#14621,#14622,#14623,#14624,#14625,#14626,#14627,#14628,
#14629,#14630,#14631,#14632,#14633,#14634,#14635,#14636,#14637,#14638,#14639,
#14640,#14641,#14642,#14643,#14644,#14645,#14646,#14647,#14648,#14649,#14650,
#14651,#14652,#14653,#14654,#14655,#14656,#14657,#14658,#14659,#14660,#14661,
#14662,#14663,#14664,#14665,#14666,#14667,#14668,#14669,#14670,#14671,#14672,
#14673,#14674,#14675,#14676,#14677,#14678,#14679));
#15950=AXIS2_PLACEMENT_3D('',#25741,#18485,#18486);
#15951=AXIS2_PLACEMENT_3D('',#25742,#18487,#18488);
#15952=AXIS2_PLACEMENT_3D('',#25756,#18491,#18492);
#15953=AXIS2_PLACEMENT_3D('',#25770,#18495,#18496);
#15954=AXIS2_PLACEMENT_3D('',#25771,#18497,#18498);
#15955=AXIS2_PLACEMENT_3D('',#25777,#18499,#18500);
#15956=AXIS2_PLACEMENT_3D('',#25781,#18501,#18502);
#15957=AXIS2_PLACEMENT_3D('',#25793,#18507,#18508);
#15958=AXIS2_PLACEMENT_3D('',#25797,#18511,#18512);
#15959=AXIS2_PLACEMENT_3D('',#25807,#18516,#18517);
#15960=AXIS2_PLACEMENT_3D('',#25821,#18520,#18521);
#15961=AXIS2_PLACEMENT_3D('',#25835,#18524,#18525);
#15962=AXIS2_PLACEMENT_3D('',#25836,#18526,#18527);
#15963=AXIS2_PLACEMENT_3D('',#25842,#18528,#18529);
#15964=AXIS2_PLACEMENT_3D('',#25846,#18530,#18531);
#15965=AXIS2_PLACEMENT_3D('',#25858,#18536,#18537);
#15966=AXIS2_PLACEMENT_3D('',#25862,#18540,#18541);
#15967=AXIS2_PLACEMENT_3D('',#25872,#18545,#18546);
#15968=AXIS2_PLACEMENT_3D('',#25886,#18549,#18550);
#15969=AXIS2_PLACEMENT_3D('',#25900,#18553,#18554);
#15970=AXIS2_PLACEMENT_3D('',#25901,#18555,#18556);
#15971=AXIS2_PLACEMENT_3D('',#25907,#18557,#18558);
#15972=AXIS2_PLACEMENT_3D('',#25911,#18559,#18560);
#15973=AXIS2_PLACEMENT_3D('',#25923,#18565,#18566);
#15974=AXIS2_PLACEMENT_3D('',#25927,#18569,#18570);
#15975=AXIS2_PLACEMENT_3D('',#25937,#18574,#18575);
#15976=AXIS2_PLACEMENT_3D('',#25951,#18578,#18579);
#15977=AXIS2_PLACEMENT_3D('',#25965,#18582,#18583);
#15978=AXIS2_PLACEMENT_3D('',#25966,#18584,#18585);
#15979=AXIS2_PLACEMENT_3D('',#25972,#18586,#18587);
#15980=AXIS2_PLACEMENT_3D('',#25976,#18588,#18589);
#15981=AXIS2_PLACEMENT_3D('',#25988,#18594,#18595);
#15982=AXIS2_PLACEMENT_3D('',#25992,#18598,#18599);
#15983=AXIS2_PLACEMENT_3D('',#26002,#18603,#18604);
#15984=AXIS2_PLACEMENT_3D('',#26015,#18607,#18608);
#15985=AXIS2_PLACEMENT_3D('',#26031,#18613,#18614);
#15986=AXIS2_PLACEMENT_3D('',#26045,#18617,#18618);
#15987=AXIS2_PLACEMENT_3D('',#26047,#18619,#18620);
#15988=AXIS2_PLACEMENT_3D('',#26048,#18621,#18622);
#15989=AXIS2_PLACEMENT_3D('',#26052,#18623,#18624);
#15990=AXIS2_PLACEMENT_3D('',#26064,#18629,#18630);
#15991=AXIS2_PLACEMENT_3D('',#26066,#18631,#18632);
#15992=AXIS2_PLACEMENT_3D('',#26075,#18633,#18634);
#15993=AXIS2_PLACEMENT_3D('',#26076,#18635,#18636);
#15994=AXIS2_PLACEMENT_3D('',#26078,#18637,#18638);
#15995=AXIS2_PLACEMENT_3D('',#26082,#18640,#18641);
#15996=AXIS2_PLACEMENT_3D('',#26086,#18643,#18644);
#15997=AXIS2_PLACEMENT_3D('',#26090,#18646,#18647);
#15998=AXIS2_PLACEMENT_3D('',#26094,#18649,#18650);
#15999=AXIS2_PLACEMENT_3D('',#26098,#18652,#18653);
#16000=AXIS2_PLACEMENT_3D('',#26102,#18655,#18656);
#16001=AXIS2_PLACEMENT_3D('',#26106,#18658,#18659);
#16002=AXIS2_PLACEMENT_3D('',#26108,#18661,#18662);
#16003=AXIS2_PLACEMENT_3D('',#26109,#18663,#18664);
#16004=AXIS2_PLACEMENT_3D('',#26110,#18665,#18666);
#16005=AXIS2_PLACEMENT_3D('',#26111,#18667,#18668);
#16006=AXIS2_PLACEMENT_3D('',#26113,#18669,#18670);
#16007=AXIS2_PLACEMENT_3D('',#26117,#18672,#18673);
#16008=AXIS2_PLACEMENT_3D('',#26121,#18675,#18676);
#16009=AXIS2_PLACEMENT_3D('',#26125,#18678,#18679);
#16010=AXIS2_PLACEMENT_3D('',#26129,#18681,#18682);
#16011=AXIS2_PLACEMENT_3D('',#26133,#18684,#18685);
#16012=AXIS2_PLACEMENT_3D('',#26137,#18687,#18688);
#16013=AXIS2_PLACEMENT_3D('',#26141,#18690,#18691);
#16014=AXIS2_PLACEMENT_3D('',#26145,#18693,#18694);
#16015=AXIS2_PLACEMENT_3D('',#26148,#18696,#18697);
#16016=AXIS2_PLACEMENT_3D('',#26149,#18698,#18699);
#16017=AXIS2_PLACEMENT_3D('',#26156,#18701,#18702);
#16018=AXIS2_PLACEMENT_3D('',#26167,#18704,#18705);
#16019=AXIS2_PLACEMENT_3D('',#26173,#18706,#18707);
#16020=AXIS2_PLACEMENT_3D('',#26177,#18708,#18709);
#16021=AXIS2_PLACEMENT_3D('',#26185,#18714,#18715);
#16022=AXIS2_PLACEMENT_3D('',#26189,#18718,#18719);
#16023=AXIS2_PLACEMENT_3D('',#26199,#18723,#18724);
#16024=AXIS2_PLACEMENT_3D('',#26210,#18726,#18727);
#16025=AXIS2_PLACEMENT_3D('',#26221,#18729,#18730);
#16026=AXIS2_PLACEMENT_3D('',#26227,#18731,#18732);
#16027=AXIS2_PLACEMENT_3D('',#26231,#18733,#18734);
#16028=AXIS2_PLACEMENT_3D('',#26243,#18739,#18740);
#16029=AXIS2_PLACEMENT_3D('',#26247,#18743,#18744);
#16030=AXIS2_PLACEMENT_3D('',#26257,#18748,#18749);
#16031=AXIS2_PLACEMENT_3D('',#26266,#18754,#18755);
#16032=AXIS2_PLACEMENT_3D('',#26272,#18759,#18760);
#16033=AXIS2_PLACEMENT_3D('',#26281,#18765,#18766);
#16034=AXIS2_PLACEMENT_3D('',#26287,#18770,#18771);
#16035=AXIS2_PLACEMENT_3D('',#26296,#18776,#18777);
#16036=AXIS2_PLACEMENT_3D('',#26302,#18781,#18782);
#16037=AXIS2_PLACEMENT_3D('',#26311,#18787,#18788);
#16038=AXIS2_PLACEMENT_3D('',#26317,#18792,#18793);
#16039=AXIS2_PLACEMENT_3D('',#26326,#18798,#18799);
#16040=AXIS2_PLACEMENT_3D('',#26332,#18803,#18804);
#16041=AXIS2_PLACEMENT_3D('',#26335,#18807,#18808);
#16042=AXIS2_PLACEMENT_3D('',#26336,#18809,#18810);
#16043=AXIS2_PLACEMENT_3D('',#26339,#18813,#18814);
#16044=AXIS2_PLACEMENT_3D('',#26340,#18815,#18816);
#16045=AXIS2_PLACEMENT_3D('',#26343,#18819,#18820);
#16046=AXIS2_PLACEMENT_3D('',#26345,#18822,#18823);
#16047=AXIS2_PLACEMENT_3D('',#26348,#18826,#18827);
#16048=AXIS2_PLACEMENT_3D('',#26349,#18828,#18829);
#16049=AXIS2_PLACEMENT_3D('',#26352,#18832,#18833);
#16050=AXIS2_PLACEMENT_3D('',#26353,#18834,#18835);
#16051=AXIS2_PLACEMENT_3D('',#26356,#18838,#18839);
#16052=AXIS2_PLACEMENT_3D('',#26357,#18840,#18841);
#16053=AXIS2_PLACEMENT_3D('',#26360,#18844,#18845);
#16054=AXIS2_PLACEMENT_3D('',#26361,#18846,#18847);
#16055=AXIS2_PLACEMENT_3D('',#26372,#18849,#18850);
#16056=AXIS2_PLACEMENT_3D('',#26383,#18852,#18853);
#16057=AXIS2_PLACEMENT_3D('',#26389,#18854,#18855);
#16058=AXIS2_PLACEMENT_3D('',#26393,#18856,#18857);
#16059=AXIS2_PLACEMENT_3D('',#26400,#18860,#18861);
#16060=AXIS2_PLACEMENT_3D('',#26402,#18863,#18864);
#16061=AXIS2_PLACEMENT_3D('',#26408,#18866,#18867);
#16062=AXIS2_PLACEMENT_3D('',#26419,#18869,#18870);
#16063=AXIS2_PLACEMENT_3D('',#26430,#18872,#18873);
#16064=AXIS2_PLACEMENT_3D('',#26436,#18874,#18875);
#16065=AXIS2_PLACEMENT_3D('',#26440,#18876,#18877);
#16066=AXIS2_PLACEMENT_3D('',#26447,#18880,#18881);
#16067=AXIS2_PLACEMENT_3D('',#26449,#18883,#18884);
#16068=AXIS2_PLACEMENT_3D('',#26455,#18886,#18887);
#16069=AXIS2_PLACEMENT_3D('',#26466,#18889,#18890);
#16070=AXIS2_PLACEMENT_3D('',#26477,#18892,#18893);
#16071=AXIS2_PLACEMENT_3D('',#26483,#18894,#18895);
#16072=AXIS2_PLACEMENT_3D('',#26487,#18896,#18897);
#16073=AXIS2_PLACEMENT_3D('',#26494,#18900,#18901);
#16074=AXIS2_PLACEMENT_3D('',#26496,#18903,#18904);
#16075=AXIS2_PLACEMENT_3D('',#26502,#18906,#18907);
#16076=AXIS2_PLACEMENT_3D('',#26513,#18909,#18910);
#16077=AXIS2_PLACEMENT_3D('',#26524,#18912,#18913);
#16078=AXIS2_PLACEMENT_3D('',#26530,#18914,#18915);
#16079=AXIS2_PLACEMENT_3D('',#26534,#18916,#18917);
#16080=AXIS2_PLACEMENT_3D('',#26541,#18920,#18921);
#16081=AXIS2_PLACEMENT_3D('',#26543,#18923,#18924);
#16082=AXIS2_PLACEMENT_3D('',#26549,#18926,#18927);
#16083=AXIS2_PLACEMENT_3D('',#26560,#18929,#18930);
#16084=AXIS2_PLACEMENT_3D('',#26571,#18932,#18933);
#16085=AXIS2_PLACEMENT_3D('',#26577,#18934,#18935);
#16086=AXIS2_PLACEMENT_3D('',#26581,#18936,#18937);
#16087=AXIS2_PLACEMENT_3D('',#26584,#18940,#18941);
#16088=AXIS2_PLACEMENT_3D('',#26590,#18943,#18944);
#16089=AXIS2_PLACEMENT_3D('',#26599,#18945,#18946);
#16090=AXIS2_PLACEMENT_3D('',#26600,#18947,#18948);
#16091=AXIS2_PLACEMENT_3D('',#26609,#18953,#18954);
#16092=AXIS2_PLACEMENT_3D('',#26615,#18958,#18959);
#16093=AXIS2_PLACEMENT_3D('',#26622,#18961,#18962);
#16094=AXIS2_PLACEMENT_3D('',#26633,#18964,#18965);
#16095=AXIS2_PLACEMENT_3D('',#26639,#18966,#18967);
#16096=AXIS2_PLACEMENT_3D('',#26643,#18968,#18969);
#16097=AXIS2_PLACEMENT_3D('',#26646,#18972,#18973);
#16098=AXIS2_PLACEMENT_3D('',#26652,#18975,#18976);
#16099=AXIS2_PLACEMENT_3D('',#26653,#18977,#18978);
#16100=AXIS2_PLACEMENT_3D('',#26654,#18979,#18980);
#16101=AXIS2_PLACEMENT_3D('',#26656,#18981,#18982);
#16102=AXIS2_PLACEMENT_3D('',#26659,#18984,#18985);
#16103=AXIS2_PLACEMENT_3D('',#26660,#18986,#18987);
#16104=AXIS2_PLACEMENT_3D('',#26663,#18989,#18990);
#16105=AXIS2_PLACEMENT_3D('',#26664,#18991,#18992);
#16106=AXIS2_PLACEMENT_3D('',#26666,#18994,#18995);
#16107=AXIS2_PLACEMENT_3D('',#26667,#18996,#18997);
#16108=AXIS2_PLACEMENT_3D('',#26668,#18998,#18999);
#16109=AXIS2_PLACEMENT_3D('',#26669,#19000,#19001);
#16110=AXIS2_PLACEMENT_3D('',#26670,#19002,#19003);
#16111=AXIS2_PLACEMENT_3D('',#26671,#19004,#19005);
#16112=AXIS2_PLACEMENT_3D('',#26672,#19006,#19007);
#16113=AXIS2_PLACEMENT_3D('',#26673,#19008,#19009);
#16114=AXIS2_PLACEMENT_3D('',#26674,#19010,#19011);
#16115=AXIS2_PLACEMENT_3D('',#26676,#19012,#19013);
#16116=AXIS2_PLACEMENT_3D('',#26678,#19015,#19016);
#16117=AXIS2_PLACEMENT_3D('',#26679,#19017,#19018);
#16118=AXIS2_PLACEMENT_3D('',#26682,#19019,#19020);
#16119=AXIS2_PLACEMENT_3D('',#26688,#19024,#19025);
#16120=AXIS2_PLACEMENT_3D('',#26694,#19029,#19030);
#16121=AXIS2_PLACEMENT_3D('',#26700,#19034,#19035);
#16122=AXIS2_PLACEMENT_3D('',#26701,#19036,#19037);
#16123=AXIS2_PLACEMENT_3D('',#26703,#19039,#19040);
#16124=AXIS2_PLACEMENT_3D('',#26704,#19041,#19042);
#16125=AXIS2_PLACEMENT_3D('',#26705,#19043,#19044);
#16126=AXIS2_PLACEMENT_3D('',#26706,#19045,#19046);
#16127=AXIS2_PLACEMENT_3D('',#26707,#19047,#19048);
#16128=AXIS2_PLACEMENT_3D('',#26708,#19049,#19050);
#16129=AXIS2_PLACEMENT_3D('',#26709,#19051,#19052);
#16130=AXIS2_PLACEMENT_3D('',#26710,#19053,#19054);
#16131=AXIS2_PLACEMENT_3D('',#26711,#19055,#19056);
#16132=AXIS2_PLACEMENT_3D('',#26712,#19057,#19058);
#16133=AXIS2_PLACEMENT_3D('',#26713,#19059,#19060);
#16134=AXIS2_PLACEMENT_3D('',#26714,#19061,#19062);
#16135=AXIS2_PLACEMENT_3D('',#26715,#19063,#19064);
#16136=AXIS2_PLACEMENT_3D('',#26719,#19065,#19066);
#16137=AXIS2_PLACEMENT_3D('',#26720,#19067,#19068);
#16138=AXIS2_PLACEMENT_3D('',#26722,#19069,#19070);
#16139=AXIS2_PLACEMENT_3D('',#26723,#19071,#19072);
#16140=AXIS2_PLACEMENT_3D('',#26725,#19073,#19074);
#16141=AXIS2_PLACEMENT_3D('',#26727,#19076,#19077);
#16142=AXIS2_PLACEMENT_3D('',#26729,#19078,#19079);
#16143=AXIS2_PLACEMENT_3D('',#26730,#19080,#19081);
#16144=AXIS2_PLACEMENT_3D('',#26732,#19082,#19083);
#16145=AXIS2_PLACEMENT_3D('',#26734,#19085,#19086);
#16146=AXIS2_PLACEMENT_3D('',#26736,#19087,#19088);
#16147=AXIS2_PLACEMENT_3D('',#26737,#19089,#19090);
#16148=AXIS2_PLACEMENT_3D('',#26739,#19091,#19092);
#16149=AXIS2_PLACEMENT_3D('',#26741,#19094,#19095);
#16150=AXIS2_PLACEMENT_3D('',#26743,#19096,#19097);
#16151=AXIS2_PLACEMENT_3D('',#26745,#19099,#19100);
#18485=DIRECTION('axis',(0.,0.,1.));
#18486=DIRECTION('refdir',(1.,0.,0.));
#18487=DIRECTION('center_axis',(0.,0.993813628552114,-0.111060666773081));
#18488=DIRECTION('ref_axis',(0.,0.111060666773081,0.993813628552114));
#18489=DIRECTION('',(-1.,0.,0.));
#18490=DIRECTION('',(1.,0.,0.));
#18491=DIRECTION('center_axis',(0.,0.248567642137747,0.968614540094294));
#18492=DIRECTION('ref_axis',(1.,0.,0.));
#18493=DIRECTION('',(-1.,0.,0.));
#18494=DIRECTION('',(1.,0.,0.));
#18495=DIRECTION('center_axis',(1.,0.,0.));
#18496=DIRECTION('ref_axis',(0.,1.,0.));
#18497=DIRECTION('center_axis',(-1.,0.,0.));
#18498=DIRECTION('ref_axis',(0.,1.,0.));
#18499=DIRECTION('center_axis',(1.,0.,0.));
#18500=DIRECTION('ref_axis',(0.,1.,0.));
#18501=DIRECTION('center_axis',(0.,-0.568064746731156,0.822983865893657));
#18502=DIRECTION('ref_axis',(0.,-0.822983865893656,-0.568064746731156));
#18503=DIRECTION('',(0.,-0.822983865893656,-0.568064746731156));
#18504=DIRECTION('',(1.,0.,0.));
#18505=DIRECTION('',(-0.707106781186546,-0.581937472380526,-0.401682434566619));
#18506=DIRECTION('',(0.,-0.822983865893656,-0.568064746731156));
#18507=DIRECTION('center_axis',(1.,0.,0.));
#18508=DIRECTION('ref_axis',(0.,-0.822983865893656,-0.568064746731156));
#18509=DIRECTION('',(0.,0.822983865893656,0.568064746731156));
#18510=DIRECTION('',(0.,0.568064746731156,-0.822983865893656));
#18511=DIRECTION('center_axis',(0.,0.568064746731156,-0.822983865893657));
#18512=DIRECTION('ref_axis',(0.,0.822983865893656,0.568064746731156));
#18513=DIRECTION('',(0.,0.822983865893656,0.568064746731156));
#18514=DIRECTION('',(0.707106781186546,0.581937472380526,0.401682434566619));
#18515=DIRECTION('',(1.,0.,0.));
#18516=DIRECTION('center_axis',(0.,0.828365800425665,-0.560187558488358));
#18517=DIRECTION('ref_axis',(-1.,0.,0.));
#18518=DIRECTION('',(-1.,0.,0.));
#18519=DIRECTION('',(1.,0.,0.));
#18520=DIRECTION('center_axis',(0.,0.670233338073619,0.742150437940108));
#18521=DIRECTION('ref_axis',(1.,0.,0.));
#18522=DIRECTION('',(-1.,0.,0.));
#18523=DIRECTION('',(1.,0.,0.));
#18524=DIRECTION('center_axis',(1.,0.,0.));
#18525=DIRECTION('ref_axis',(0.,1.,0.));
#18526=DIRECTION('center_axis',(-1.,0.,0.));
#18527=DIRECTION('ref_axis',(0.,1.,0.));
#18528=DIRECTION('center_axis',(1.,0.,0.));
#18529=DIRECTION('ref_axis',(0.,1.,0.));
#18530=DIRECTION('center_axis',(0.,-0.120536680255322,0.992708874098054));
#18531=DIRECTION('ref_axis',(0.,-0.992708874098054,-0.120536680255322));
#18532=DIRECTION('',(0.,-0.992708874098054,-0.120536680255322));
#18533=DIRECTION('',(1.,0.,0.));
#18534=DIRECTION('',(-0.707106781186546,-0.701951176618798,-0.0852323039902532));
#18535=DIRECTION('',(0.,-0.992708874098054,-0.120536680255322));
#18536=DIRECTION('center_axis',(1.,0.,0.));
#18537=DIRECTION('ref_axis',(0.,-0.992708874098054,-0.120536680255322));
#18538=DIRECTION('',(0.,0.992708874098054,0.120536680255322));
#18539=DIRECTION('',(0.,0.120536680255322,-0.992708874098054));
#18540=DIRECTION('center_axis',(0.,0.120536680255322,-0.992708874098054));
#18541=DIRECTION('ref_axis',(0.,0.992708874098054,0.120536680255322));
#18542=DIRECTION('',(0.,0.992708874098054,0.120536680255322));
#18543=DIRECTION('',(0.707106781186546,0.701951176618798,0.0852323039902532));
#18544=DIRECTION('',(1.,0.,0.));
#18545=DIRECTION('center_axis',(0.,0.473149350311789,-0.880982231545865));
#18546=DIRECTION('ref_axis',(-1.,0.,0.));
#18547=DIRECTION('',(-1.,0.,0.));
#18548=DIRECTION('',(1.,0.,0.));
#18549=DIRECTION('center_axis',(0.,0.938356653444149,0.345668614336183));
#18550=DIRECTION('ref_axis',(0.,-0.345668614336183,0.938356653444149));
#18551=DIRECTION('',(-1.,0.,0.));
#18552=DIRECTION('',(1.,0.,0.));
#18553=DIRECTION('center_axis',(1.,0.,0.));
#18554=DIRECTION('ref_axis',(0.,1.,0.));
#18555=DIRECTION('center_axis',(-1.,0.,0.));
#18556=DIRECTION('ref_axis',(0.,1.,0.));
#18557=DIRECTION('center_axis',(1.,0.,0.));
#18558=DIRECTION('ref_axis',(0.,1.,0.));
#18559=DIRECTION('center_axis',(0.,0.354604887042536,0.935016242685415));
#18560=DIRECTION('ref_axis',(0.,-0.935016242685415,0.354604887042536));
#18561=DIRECTION('',(0.,-0.935016242685415,0.354604887042536));
#18562=DIRECTION('',(1.,0.,0.));
#18563=DIRECTION('',(-0.707106781186546,-0.661156325722425,0.250743520269667));
#18564=DIRECTION('',(0.,-0.935016242685415,0.354604887042536));
#18565=DIRECTION('center_axis',(1.,0.,0.));
#18566=DIRECTION('ref_axis',(0.,-0.935016242685415,0.354604887042536));
#18567=DIRECTION('',(0.,0.935016242685415,-0.354604887042536));
#18568=DIRECTION('',(0.,-0.354604887042536,-0.935016242685415));
#18569=DIRECTION('center_axis',(0.,-0.354604887042536,-0.935016242685415));
#18570=DIRECTION('ref_axis',(0.,0.935016242685415,-0.354604887042536));
#18571=DIRECTION('',(0.,0.935016242685415,-0.354604887042536));
#18572=DIRECTION('',(0.707106781186546,0.661156325722425,-0.250743520269667));
#18573=DIRECTION('',(1.,0.,0.));
#18574=DIRECTION('center_axis',(0.,0.00954008610927885,-0.99995449234304));
#18575=DIRECTION('ref_axis',(-1.,0.,0.));
#18576=DIRECTION('',(-1.,0.,0.));
#18577=DIRECTION('',(1.,0.,0.));
#18578=DIRECTION('center_axis',(0.,0.991513767934188,-0.130001723053771));
#18579=DIRECTION('ref_axis',(0.,0.130001723053771,0.991513767934188));
#18580=DIRECTION('',(-1.,0.,0.));
#18581=DIRECTION('',(1.,0.,0.));
#18582=DIRECTION('center_axis',(1.,0.,0.));
#18583=DIRECTION('ref_axis',(0.,1.,0.));
#18584=DIRECTION('center_axis',(-1.,0.,0.));
#18585=DIRECTION('ref_axis',(0.,1.,0.));
#18586=DIRECTION('center_axis',(1.,0.,0.));
#18587=DIRECTION('ref_axis',(0.,1.,0.));
#18588=DIRECTION('center_axis',(0.,0.748510748171101,0.663122658240795));
#18589=DIRECTION('ref_axis',(0.,-0.663122658240795,0.748510748171101));
#18590=DIRECTION('',(0.,-0.663122658240795,0.748510748171101));
#18591=DIRECTION('',(1.,0.,0.));
#18592=DIRECTION('',(-0.707106781186547,-0.468898528400516,0.529277025822802));
#18593=DIRECTION('',(0.,-0.663122658240795,0.748510748171101));
#18594=DIRECTION('center_axis',(1.,0.,0.));
#18595=DIRECTION('ref_axis',(0.,-0.663122658240795,0.748510748171101));
#18596=DIRECTION('',(0.,0.663122658240795,-0.748510748171101));
#18597=DIRECTION('',(0.,-0.748510748171101,-0.663122658240795));
#18598=DIRECTION('center_axis',(0.,-0.748510748171101,-0.663122658240795));
#18599=DIRECTION('ref_axis',(0.,0.663122658240795,-0.748510748171101));
#18600=DIRECTION('',(0.,0.663122658240795,-0.748510748171101));
#18601=DIRECTION('',(0.707106781186547,0.468898528400516,-0.529277025822802));
#18602=DIRECTION('',(1.,0.,0.));
#18603=DIRECTION('center_axis',(0.,-0.456254696850359,-0.889849229702418));
#18604=DIRECTION('ref_axis',(-1.,0.,0.));
#18605=DIRECTION('',(1.,0.,0.));
#18606=DIRECTION('',(-1.,0.,0.));
#18607=DIRECTION('center_axis',(0.,0.970941817426052,0.239315664287557));
#18608=DIRECTION('ref_axis',(0.,-0.239315664287557,0.970941817426052));
#18609=DIRECTION('',(0.,-0.239315664287557,0.970941817426052));
#18610=DIRECTION('',(1.,0.,0.));
#18611=DIRECTION('',(-0.707106781186546,-0.169221729061895,0.686559543239553));
#18612=DIRECTION('',(0.,-0.239315664287557,0.970941817426052));
#18613=DIRECTION('center_axis',(0.,0.817527027226742,-0.575890232382705));
#18614=DIRECTION('ref_axis',(-1.,0.,0.));
#18615=DIRECTION('',(-1.,0.,0.));
#18616=DIRECTION('',(1.,0.,0.));
#18617=DIRECTION('center_axis',(1.,0.,0.));
#18618=DIRECTION('ref_axis',(0.,1.,0.));
#18619=DIRECTION('center_axis',(1.,0.,0.));
#18620=DIRECTION('ref_axis',(0.,1.,0.));
#18621=DIRECTION('center_axis',(-1.,0.,0.));
#18622=DIRECTION('ref_axis',(0.,1.,0.));
#18623=DIRECTION('center_axis',(0.,-0.970941817426052,-0.239315664287557));
#18624=DIRECTION('ref_axis',(0.,0.239315664287557,-0.970941817426052));
#18625=DIRECTION('',(0.,0.239315664287557,-0.970941817426052));
#18626=DIRECTION('',(0.707106781186546,0.169221729061895,-0.686559543239553));
#18627=DIRECTION('',(1.,0.,0.));
#18628=DIRECTION('',(0.,0.239315664287557,-0.970941817426052));
#18629=DIRECTION('center_axis',(1.,0.,0.));
#18630=DIRECTION('ref_axis',(0.,1.,0.));
#18631=DIRECTION('center_axis',(1.,0.,0.));
#18632=DIRECTION('ref_axis',(0.,0.,-1.));
#18633=DIRECTION('center_axis',(1.,0.,0.));
#18634=DIRECTION('ref_axis',(0.,0.,-1.));
#18635=DIRECTION('center_axis',(1.,0.,0.));
#18636=DIRECTION('ref_axis',(0.,1.,0.));
#18637=DIRECTION('center_axis',(1.,0.,0.));
#18638=DIRECTION('ref_axis',(0.,0.,-1.));
#18639=DIRECTION('',(-1.,0.,0.));
#18640=DIRECTION('center_axis',(-1.,0.,0.));
#18641=DIRECTION('ref_axis',(0.,-1.,0.));
#18642=DIRECTION('',(1.,0.,0.));
#18643=DIRECTION('center_axis',(1.,0.,0.));
#18644=DIRECTION('ref_axis',(0.,0.,-1.));
#18645=DIRECTION('',(-1.,0.,0.));
#18646=DIRECTION('center_axis',(-1.,0.,0.));
#18647=DIRECTION('ref_axis',(0.,-1.,0.));
#18648=DIRECTION('',(1.,0.,0.));
#18649=DIRECTION('center_axis',(1.,0.,0.));
#18650=DIRECTION('ref_axis',(0.,0.,-1.));
#18651=DIRECTION('',(-1.,0.,0.));
#18652=DIRECTION('center_axis',(-1.,0.,0.));
#18653=DIRECTION('ref_axis',(0.,-1.,0.));
#18654=DIRECTION('',(1.,0.,0.));
#18655=DIRECTION('center_axis',(1.,0.,0.));
#18656=DIRECTION('ref_axis',(0.,0.,-1.));
#18657=DIRECTION('',(-1.,0.,0.));
#18658=DIRECTION('center_axis',(-1.,0.,0.));
#18659=DIRECTION('ref_axis',(0.,-1.,0.));
#18660=DIRECTION('',(1.,0.,0.));
#18661=DIRECTION('center_axis',(1.,0.,0.));
#18662=DIRECTION('ref_axis',(0.,0.,-1.));
#18663=DIRECTION('center_axis',(1.,0.,0.));
#18664=DIRECTION('ref_axis',(0.,0.,-1.));
#18665=DIRECTION('center_axis',(1.,0.,0.));
#18666=DIRECTION('ref_axis',(0.,0.,-1.));
#18667=DIRECTION('center_axis',(1.,0.,0.));
#18668=DIRECTION('ref_axis',(0.,0.,-1.));
#18669=DIRECTION('center_axis',(1.,0.,0.));
#18670=DIRECTION('ref_axis',(0.,0.,-1.));
#18671=DIRECTION('',(-1.,0.,0.));
#18672=DIRECTION('center_axis',(-1.,0.,0.));
#18673=DIRECTION('ref_axis',(0.,1.,0.));
#18674=DIRECTION('',(1.,0.,0.));
#18675=DIRECTION('center_axis',(1.,0.,0.));
#18676=DIRECTION('ref_axis',(0.,0.,-1.));
#18677=DIRECTION('',(-1.,0.,0.));
#18678=DIRECTION('center_axis',(-1.,0.,0.));
#18679=DIRECTION('ref_axis',(0.,1.,0.));
#18680=DIRECTION('',(1.,0.,0.));
#18681=DIRECTION('center_axis',(1.,0.,0.));
#18682=DIRECTION('ref_axis',(0.,0.,-1.));
#18683=DIRECTION('',(-1.,0.,0.));
#18684=DIRECTION('center_axis',(-1.,0.,0.));
#18685=DIRECTION('ref_axis',(0.,-1.,0.));
#18686=DIRECTION('',(1.,0.,0.));
#18687=DIRECTION('center_axis',(1.,0.,0.));
#18688=DIRECTION('ref_axis',(0.,0.,-1.));
#18689=DIRECTION('',(-1.,0.,0.));
#18690=DIRECTION('center_axis',(-1.,0.,0.));
#18691=DIRECTION('ref_axis',(0.,-1.,0.));
#18692=DIRECTION('',(1.,0.,0.));
#18693=DIRECTION('center_axis',(1.,0.,0.));
#18694=DIRECTION('ref_axis',(0.,0.,-1.));
#18695=DIRECTION('',(-1.,0.,0.));
#18696=DIRECTION('center_axis',(-1.,0.,0.));
#18697=DIRECTION('ref_axis',(0.,-1.,0.));
#18698=DIRECTION('center_axis',(0.,-0.817527027226745,-0.575890232382701));
#18699=DIRECTION('ref_axis',(-1.,0.,0.));
#18700=DIRECTION('',(-1.,0.,0.));
#18701=DIRECTION('center_axis',(0.,0.456254696850359,-0.889849229702418));
#18702=DIRECTION('ref_axis',(-1.,0.,0.));
#18703=DIRECTION('',(1.,0.,0.));
#18704=DIRECTION('center_axis',(1.,0.,0.));
#18705=DIRECTION('ref_axis',(0.,-1.,0.));
#18706=DIRECTION('center_axis',(1.,0.,0.));
#18707=DIRECTION('ref_axis',(0.,-1.,0.));
#18708=DIRECTION('center_axis',(0.,0.970941817426052,-0.239315664287558));
#18709=DIRECTION('ref_axis',(0.,0.239315664287558,0.970941817426052));
#18710=DIRECTION('',(0.,0.239315664287558,0.970941817426052));
#18711=DIRECTION('',(1.,0.,0.));
#18712=DIRECTION('',(-0.707106781186545,0.169221729061896,0.686559543239555));
#18713=DIRECTION('',(0.,0.239315664287558,0.970941817426052));
#18714=DIRECTION('center_axis',(1.,0.,0.));
#18715=DIRECTION('ref_axis',(0.,0.239315664287558,0.970941817426052));
#18716=DIRECTION('',(0.,-0.239315664287558,-0.970941817426052));
#18717=DIRECTION('',(0.,-0.970941817426052,0.239315664287558));
#18718=DIRECTION('center_axis',(0.,-0.970941817426052,0.239315664287558));
#18719=DIRECTION('ref_axis',(0.,-0.239315664287558,-0.970941817426052));
#18720=DIRECTION('',(0.,-0.239315664287558,-0.970941817426052));
#18721=DIRECTION('',(0.707106781186545,-0.169221729061896,-0.686559543239555));
#18722=DIRECTION('',(1.,0.,0.));
#18723=DIRECTION('center_axis',(0.,-0.991513767934189,-0.130001723053764));
#18724=DIRECTION('ref_axis',(0.,0.130001723053764,-0.991513767934189));
#18725=DIRECTION('',(-1.,0.,0.));
#18726=DIRECTION('center_axis',(0.,-0.00954008610928227,-0.99995449234304));
#18727=DIRECTION('ref_axis',(-1.,0.,0.));
#18728=DIRECTION('',(1.,0.,0.));
#18729=DIRECTION('center_axis',(1.,0.,0.));
#18730=DIRECTION('ref_axis',(0.,-1.,0.));
#18731=DIRECTION('center_axis',(1.,0.,0.));
#18732=DIRECTION('ref_axis',(0.,-1.,0.));
#18733=DIRECTION('center_axis',(0.,0.748510748171101,-0.663122658240796));
#18734=DIRECTION('ref_axis',(0.,0.663122658240796,0.748510748171101));
#18735=DIRECTION('',(0.,0.663122658240796,0.748510748171101));
#18736=DIRECTION('',(1.,0.,0.));
#18737=DIRECTION('',(-0.707106781186547,0.468898528400516,0.529277025822802));
#18738=DIRECTION('',(0.,0.663122658240796,0.748510748171101));
#18739=DIRECTION('center_axis',(1.,0.,0.));
#18740=DIRECTION('ref_axis',(0.,0.663122658240796,0.748510748171101));
#18741=DIRECTION('',(0.,-0.663122658240796,-0.748510748171101));
#18742=DIRECTION('',(0.,-0.748510748171101,0.663122658240796));
#18743=DIRECTION('center_axis',(0.,-0.748510748171101,0.663122658240796));
#18744=DIRECTION('ref_axis',(0.,-0.663122658240796,-0.748510748171101));
#18745=DIRECTION('',(0.,-0.663122658240796,-0.748510748171101));
#18746=DIRECTION('',(0.707106781186547,-0.468898528400516,-0.529277025822802));
#18747=DIRECTION('',(1.,0.,0.));
#18748=DIRECTION('center_axis',(-0.707106781186549,0.,0.707106781186546));
#18749=DIRECTION('ref_axis',(0.707106781186546,0.,0.707106781186549));
#18750=DIRECTION('',(-0.707106781186546,0.,-0.707106781186549));
#18751=DIRECTION('',(0.,1.,0.));
#18752=DIRECTION('',(0.707106781186546,0.,0.707106781186549));
#18753=DIRECTION('',(0.,-1.,0.));
#18754=DIRECTION('center_axis',(0.,0.,-1.));
#18755=DIRECTION('ref_axis',(0.,1.,0.));
#18756=DIRECTION('',(1.,0.,0.));
#18757=DIRECTION('',(0.,1.,0.));
#18758=DIRECTION('',(1.,0.,0.));
#18759=DIRECTION('center_axis',(-0.707106781186548,-0.328608906326671,0.626111960181874));
#18760=DIRECTION('ref_axis',(0.662926885132466,0.,0.748684142324763));
#18761=DIRECTION('',(-0.707106781186547,0.328608906326672,-0.626111960181875));
#18762=DIRECTION('',(0.,0.88545602565321,0.464723172043769));
#18763=DIRECTION('',(0.707106781186547,-0.328608906326672,0.626111960181875));
#18764=DIRECTION('',(0.,-0.88545602565321,-0.464723172043769));
#18765=DIRECTION('center_axis',(0.,0.464723172043769,-0.88545602565321));
#18766=DIRECTION('ref_axis',(0.,0.88545602565321,0.464723172043769));
#18767=DIRECTION('',(1.,0.,0.));
#18768=DIRECTION('',(0.,0.88545602565321,0.464723172043769));
#18769=DIRECTION('',(1.,0.,0.));
#18770=DIRECTION('center_axis',(-0.707106781186548,-0.581937472380525,0.401682434566619));
#18771=DIRECTION('ref_axis',(0.493932454279441,0.,0.869500276371139));
#18772=DIRECTION('',(-0.707106781186547,0.581937472380525,-0.401682434566619));
#18773=DIRECTION('',(0.,0.568064746731156,0.822983865893656));
#18774=DIRECTION('',(0.707106781186547,-0.581937472380525,0.401682434566619));
#18775=DIRECTION('',(0.,-0.568064746731156,-0.822983865893656));
#18776=DIRECTION('center_axis',(0.,0.822983865893656,-0.568064746731156));
#18777=DIRECTION('ref_axis',(0.,0.568064746731156,0.822983865893656));
#18778=DIRECTION('',(1.,0.,0.));
#18779=DIRECTION('',(0.,0.568064746731156,0.822983865893656));
#18780=DIRECTION('',(1.,0.,0.));
#18781=DIRECTION('center_axis',(-0.707106781186548,-0.701951176618796,0.0852323039902536));
#18782=DIRECTION('ref_axis',(0.119670463698395,0.,0.992813668378015));
#18783=DIRECTION('',(-0.707106781186547,0.701951176618797,-0.0852323039902537));
#18784=DIRECTION('',(0.,0.120536680255323,0.992708874098054));
#18785=DIRECTION('',(0.707106781186547,-0.701951176618797,0.0852323039902537));
#18786=DIRECTION('',(0.,-0.120536680255323,-0.992708874098054));
#18787=DIRECTION('center_axis',(0.,0.992708874098054,-0.120536680255323));
#18788=DIRECTION('ref_axis',(0.,0.120536680255323,0.992708874098054));
#18789=DIRECTION('',(1.,0.,0.));
#18790=DIRECTION('',(0.,0.120536680255323,0.992708874098054));
#18791=DIRECTION('',(1.,0.,0.));
#18792=DIRECTION('center_axis',(-0.707106781186548,-0.661156325722423,-0.250743520269666));
#18793=DIRECTION('ref_axis',(-0.33421410555183,0.,0.942497178590042));
#18794=DIRECTION('',(-0.707106781186547,0.661156325722424,0.250743520269667));
#18795=DIRECTION('',(0.,-0.354604887042536,0.935016242685415));
#18796=DIRECTION('',(0.707106781186547,-0.661156325722424,-0.250743520269667));
#18797=DIRECTION('',(0.,0.354604887042536,-0.935016242685415));
#18798=DIRECTION('center_axis',(0.,0.935016242685415,0.354604887042536));
#18799=DIRECTION('ref_axis',(0.,-0.354604887042536,0.935016242685415));
#18800=DIRECTION('',(1.,0.,0.));
#18801=DIRECTION('',(0.,-0.354604887042536,0.935016242685415));
#18802=DIRECTION('',(1.,0.,0.));
#18803=DIRECTION('center_axis',(-0.707106781186548,-0.468898528400515,-0.529277025822801));
#18804=DIRECTION('ref_axis',(-0.59923668503494,0.,0.800571917636596));
#18805=DIRECTION('',(0.,-0.748510748171101,0.663122658240796));
#18806=DIRECTION('',(0.,0.748510748171101,-0.663122658240796));
#18807=DIRECTION('center_axis',(0.,0.663122658240796,0.748510748171101));
#18808=DIRECTION('ref_axis',(0.,-0.748510748171101,0.663122658240796));
#18809=DIRECTION('center_axis',(-0.70710678118655,-0.169221729061895,-0.686559543239549));
#18810=DIRECTION('ref_axis',(-0.696605990477037,0.,0.717453896798607));
#18811=DIRECTION('',(0.,-0.970941817426052,0.239315664287558));
#18812=DIRECTION('',(0.,0.970941817426052,-0.239315664287558));
#18813=DIRECTION('center_axis',(0.,0.239315664287558,0.970941817426052));
#18814=DIRECTION('ref_axis',(0.,-0.970941817426052,0.239315664287558));
#18815=DIRECTION('center_axis',(-0.707106781186549,0.169221729061895,-0.686559543239551));
#18816=DIRECTION('ref_axis',(-0.696605990477039,0.,0.717453896798605));
#18817=DIRECTION('',(0.,-0.970941817426052,-0.239315664287557));
#18818=DIRECTION('',(0.,0.970941817426052,0.239315664287557));
#18819=DIRECTION('center_axis',(0.,-0.239315664287557,0.970941817426052));
#18820=DIRECTION('ref_axis',(0.,-0.970941817426052,-0.239315664287557));
#18821=DIRECTION('',(0.,-0.970941817426052,-0.239315664287557));
#18822=DIRECTION('center_axis',(-0.707106781186548,0.468898528400515,-0.529277025822801));
#18823=DIRECTION('ref_axis',(-0.59923668503494,0.,0.800571917636595));
#18824=DIRECTION('',(0.,-0.748510748171101,-0.663122658240795));
#18825=DIRECTION('',(0.,0.748510748171101,0.663122658240795));
#18826=DIRECTION('center_axis',(0.,-0.663122658240795,0.748510748171101));
#18827=DIRECTION('ref_axis',(0.,-0.748510748171101,-0.663122658240795));
#18828=DIRECTION('center_axis',(-0.707106781186549,0.661156325722422,-0.250743520269666));
#18829=DIRECTION('ref_axis',(-0.334214105551829,0.,0.942497178590043));
#18830=DIRECTION('',(0.,-0.354604887042536,-0.935016242685415));
#18831=DIRECTION('',(0.,0.354604887042536,0.935016242685415));
#18832=DIRECTION('center_axis',(0.,-0.935016242685415,0.354604887042536));
#18833=DIRECTION('ref_axis',(0.,-0.354604887042536,-0.935016242685415));
#18834=DIRECTION('center_axis',(-0.707106781186549,0.701951176618796,0.0852323039902529));
#18835=DIRECTION('ref_axis',(0.119670463698394,0.,0.992813668378015));
#18836=DIRECTION('',(0.,0.120536680255322,-0.992708874098054));
#18837=DIRECTION('',(0.,-0.120536680255322,0.992708874098054));
#18838=DIRECTION('center_axis',(0.,-0.992708874098054,-0.120536680255322));
#18839=DIRECTION('ref_axis',(0.,0.120536680255322,-0.992708874098054));
#18840=DIRECTION('center_axis',(-0.707106781186549,0.581937472380524,0.401682434566618));
#18841=DIRECTION('ref_axis',(0.49393245427944,0.,0.86950027637114));
#18842=DIRECTION('',(0.,0.568064746731156,-0.822983865893656));
#18843=DIRECTION('',(0.,-0.568064746731156,0.822983865893656));
#18844=DIRECTION('center_axis',(0.,-0.822983865893657,-0.568064746731156));
#18845=DIRECTION('ref_axis',(0.,0.568064746731156,-0.822983865893656));
#18846=DIRECTION('center_axis',(0.,-0.938356653444149,0.345668614336183));
#18847=DIRECTION('ref_axis',(0.,-0.345668614336183,-0.938356653444149));
#18848=DIRECTION('',(-1.,0.,0.));
#18849=DIRECTION('center_axis',(0.,-0.473149350311788,-0.880982231545865));
#18850=DIRECTION('ref_axis',(-1.,0.,0.));
#18851=DIRECTION('',(1.,0.,0.));
#18852=DIRECTION('center_axis',(1.,0.,0.));
#18853=DIRECTION('ref_axis',(0.,-1.,0.));
#18854=DIRECTION('center_axis',(1.,0.,0.));
#18855=DIRECTION('ref_axis',(0.,-1.,0.));
#18856=DIRECTION('center_axis',(0.,0.354604887042536,-0.935016242685415));
#18857=DIRECTION('ref_axis',(0.,0.935016242685415,0.354604887042536));
#18858=DIRECTION('',(0.,0.935016242685415,0.354604887042536));
#18859=DIRECTION('',(0.,0.935016242685415,0.354604887042536));
#18860=DIRECTION('center_axis',(1.,0.,0.));
#18861=DIRECTION('ref_axis',(0.,0.935016242685415,0.354604887042536));
#18862=DIRECTION('',(0.,-0.935016242685415,-0.354604887042536));
#18863=DIRECTION('center_axis',(0.,-0.354604887042536,0.935016242685415));
#18864=DIRECTION('ref_axis',(0.,-0.935016242685415,-0.354604887042536));
#18865=DIRECTION('',(0.,-0.935016242685415,-0.354604887042536));
#18866=DIRECTION('center_axis',(0.,-0.670233338073617,0.742150437940109));
#18867=DIRECTION('ref_axis',(1.,0.,0.));
#18868=DIRECTION('',(-1.,0.,0.));
#18869=DIRECTION('center_axis',(0.,-0.828365800425666,-0.560187558488357));
#18870=DIRECTION('ref_axis',(-1.,0.,0.));
#18871=DIRECTION('',(1.,0.,0.));
#18872=DIRECTION('center_axis',(1.,0.,0.));
#18873=DIRECTION('ref_axis',(0.,-1.,0.));
#18874=DIRECTION('center_axis',(1.,0.,0.));
#18875=DIRECTION('ref_axis',(0.,-1.,0.));
#18876=DIRECTION('center_axis',(0.,-0.120536680255323,-0.992708874098054));
#18877=DIRECTION('ref_axis',(0.,0.992708874098054,-0.120536680255323));
#18878=DIRECTION('',(0.,0.992708874098054,-0.120536680255323));
#18879=DIRECTION('',(0.,0.992708874098054,-0.120536680255323));
#18880=DIRECTION('center_axis',(1.,0.,0.));
#18881=DIRECTION('ref_axis',(0.,0.992708874098054,-0.120536680255323));
#18882=DIRECTION('',(0.,-0.992708874098054,0.120536680255323));
#18883=DIRECTION('center_axis',(0.,0.120536680255323,0.992708874098054));
#18884=DIRECTION('ref_axis',(0.,-0.992708874098054,0.120536680255323));
#18885=DIRECTION('',(0.,-0.992708874098054,0.120536680255323));
#18886=DIRECTION('center_axis',(0.,-0.248567642137749,0.968614540094294));
#18887=DIRECTION('ref_axis',(1.,0.,0.));
#18888=DIRECTION('',(-1.,0.,0.));
#18889=DIRECTION('center_axis',(0.,-0.993813628552114,-0.111060666773083));
#18890=DIRECTION('ref_axis',(0.,0.111060666773083,-0.993813628552114));
#18891=DIRECTION('',(1.,0.,0.));
#18892=DIRECTION('center_axis',(1.,0.,0.));
#18893=DIRECTION('ref_axis',(0.,-1.,0.));
#18894=DIRECTION('center_axis',(1.,0.,0.));
#18895=DIRECTION('ref_axis',(0.,-1.,0.));
#18896=DIRECTION('center_axis',(0.,-0.568064746731156,-0.822983865893656));
#18897=DIRECTION('ref_axis',(0.,0.822983865893656,-0.568064746731156));
#18898=DIRECTION('',(0.,0.822983865893656,-0.568064746731156));
#18899=DIRECTION('',(0.,0.822983865893656,-0.568064746731156));
#18900=DIRECTION('center_axis',(1.,0.,0.));
#18901=DIRECTION('ref_axis',(0.,0.822983865893656,-0.568064746731156));
#18902=DIRECTION('',(0.,-0.822983865893656,0.568064746731156));
#18903=DIRECTION('center_axis',(0.,0.568064746731156,0.822983865893656));
#18904=DIRECTION('ref_axis',(0.,-0.822983865893656,0.568064746731156));
#18905=DIRECTION('',(0.,-0.822983865893656,0.568064746731156));
#18906=DIRECTION('center_axis',(0.,0.230041905047053,0.9731807241835));
#18907=DIRECTION('ref_axis',(1.,0.,0.));
#18908=DIRECTION('',(-1.,0.,0.));
#18909=DIRECTION('center_axis',(0.,-0.931590731129833,0.363508885273776));
#18910=DIRECTION('ref_axis',(0.,-0.363508885273776,-0.931590731129833));
#18911=DIRECTION('',(1.,0.,0.));
#18912=DIRECTION('center_axis',(1.,0.,0.));
#18913=DIRECTION('ref_axis',(0.,-1.,0.));
#18914=DIRECTION('center_axis',(1.,0.,0.));
#18915=DIRECTION('ref_axis',(0.,-1.,0.));
#18916=DIRECTION('center_axis',(0.,-0.88545602565321,-0.464723172043769));
#18917=DIRECTION('ref_axis',(0.,0.464723172043769,-0.88545602565321));
#18918=DIRECTION('',(0.,0.464723172043769,-0.88545602565321));
#18919=DIRECTION('',(0.,0.464723172043769,-0.88545602565321));
#18920=DIRECTION('center_axis',(1.,0.,0.));
#18921=DIRECTION('ref_axis',(0.,0.464723172043769,-0.88545602565321));
#18922=DIRECTION('',(0.,-0.464723172043769,0.88545602565321));
#18923=DIRECTION('center_axis',(0.,0.88545602565321,0.464723172043769));
#18924=DIRECTION('ref_axis',(0.,-0.464723172043769,0.88545602565321));
#18925=DIRECTION('',(0.,-0.464723172043769,0.88545602565321));
#18926=DIRECTION('center_axis',(0.,0.655951624091067,0.754802932461375));
#18927=DIRECTION('ref_axis',(1.,0.,0.));
#18928=DIRECTION('',(-1.,0.,0.));
#18929=DIRECTION('center_axis',(0.,-0.655951624091067,0.754802932461375));
#18930=DIRECTION('ref_axis',(1.,0.,0.));
#18931=DIRECTION('',(1.,0.,0.));
#18932=DIRECTION('center_axis',(1.,0.,0.));
#18933=DIRECTION('ref_axis',(0.,1.,0.));
#18934=DIRECTION('center_axis',(1.,0.,0.));
#18935=DIRECTION('ref_axis',(0.,1.,0.));
#18936=DIRECTION('center_axis',(1.,0.,0.));
#18937=DIRECTION('ref_axis',(0.,0.,-1.));
#18938=DIRECTION('',(0.,0.,1.));
#18939=DIRECTION('',(0.,0.,-1.));
#18940=DIRECTION('center_axis',(0.,1.,0.));
#18941=DIRECTION('ref_axis',(0.,0.,1.));
#18942=DIRECTION('',(0.,0.,1.));
#18943=DIRECTION('center_axis',(1.,0.,0.));
#18944=DIRECTION('ref_axis',(0.,1.,0.));
#18945=DIRECTION('center_axis',(1.,0.,0.));
#18946=DIRECTION('ref_axis',(0.,0.,-1.));
#18947=DIRECTION('center_axis',(-0.707106781186548,0.328608906326671,0.626111960181873));
#18948=DIRECTION('ref_axis',(0.662926885132466,0.,0.748684142324764));
#18949=DIRECTION('',(-0.707106781186547,-0.328608906326672,-0.626111960181875));
#18950=DIRECTION('',(0.,0.88545602565321,-0.464723172043769));
#18951=DIRECTION('',(0.707106781186547,0.328608906326672,0.626111960181875));
#18952=DIRECTION('',(0.,-0.88545602565321,0.464723172043769));
#18953=DIRECTION('center_axis',(0.,-0.464723172043769,-0.88545602565321));
#18954=DIRECTION('ref_axis',(0.,0.88545602565321,-0.464723172043769));
#18955=DIRECTION('',(1.,0.,0.));
#18956=DIRECTION('',(0.,0.88545602565321,-0.464723172043769));
#18957=DIRECTION('',(1.,0.,0.));
#18958=DIRECTION('center_axis',(0.,0.931590731129832,0.363508885273778));
#18959=DIRECTION('ref_axis',(0.,-0.363508885273778,0.931590731129832));
#18960=DIRECTION('',(-1.,0.,0.));
#18961=DIRECTION('center_axis',(0.,-0.230041905047054,0.9731807241835));
#18962=DIRECTION('ref_axis',(1.,0.,0.));
#18963=DIRECTION('',(1.,0.,0.));
#18964=DIRECTION('center_axis',(1.,0.,0.));
#18965=DIRECTION('ref_axis',(0.,1.,0.));
#18966=DIRECTION('center_axis',(1.,0.,0.));
#18967=DIRECTION('ref_axis',(0.,1.,0.));
#18968=DIRECTION('center_axis',(1.,0.,0.));
#18969=DIRECTION('ref_axis',(0.,-0.464723172043769,-0.88545602565321));
#18970=DIRECTION('',(0.,0.464723172043769,0.88545602565321));
#18971=DIRECTION('',(0.,-0.464723172043769,-0.88545602565321));
#18972=DIRECTION('center_axis',(0.,0.88545602565321,-0.464723172043769));
#18973=DIRECTION('ref_axis',(0.,0.464723172043769,0.88545602565321));
#18974=DIRECTION('',(0.,0.464723172043769,0.88545602565321));
#18975=DIRECTION('center_axis',(1.,0.,0.));
#18976=DIRECTION('ref_axis',(0.,1.,0.));
#18977=DIRECTION('center_axis',(1.,0.,0.));
#18978=DIRECTION('ref_axis',(0.,0.,-1.));
#18979=DIRECTION('center_axis',(-1.,0.,0.));
#18980=DIRECTION('ref_axis',(0.,0.,-1.));
#18981=DIRECTION('center_axis',(-1.,0.,0.));
#18982=DIRECTION('ref_axis',(0.,0.,-1.));
#18983=DIRECTION('',(0.707106781186546,-8.65956056235495E-17,-0.707106781186549));
#18984=DIRECTION('center_axis',(1.,0.,0.));
#18985=DIRECTION('ref_axis',(0.,0.,-1.));
#18986=DIRECTION('center_axis',(1.,0.,0.));
#18987=DIRECTION('ref_axis',(0.,0.,-1.));
#18988=DIRECTION('',(1.,0.,0.));
#18989=DIRECTION('center_axis',(1.,0.,0.));
#18990=DIRECTION('ref_axis',(0.,0.,-1.));
#18991=DIRECTION('center_axis',(-1.,0.,0.));
#18992=DIRECTION('ref_axis',(0.,0.,1.));
#18993=DIRECTION('',(0.,-0.464723172043769,-0.88545602565321));
#18994=DIRECTION('center_axis',(1.,0.,0.));
#18995=DIRECTION('ref_axis',(0.,0.,-1.));
#18996=DIRECTION('center_axis',(1.,0.,0.));
#18997=DIRECTION('ref_axis',(0.,0.,-1.));
#18998=DIRECTION('center_axis',(1.,0.,0.));
#18999=DIRECTION('ref_axis',(0.,0.,-1.));
#19000=DIRECTION('center_axis',(1.,0.,0.));
#19001=DIRECTION('ref_axis',(0.,0.,-1.));
#19002=DIRECTION('center_axis',(1.,0.,0.));
#19003=DIRECTION('ref_axis',(0.,0.,-1.));
#19004=DIRECTION('center_axis',(1.,0.,0.));
#19005=DIRECTION('ref_axis',(0.,0.,-1.));
#19006=DIRECTION('center_axis',(1.,0.,0.));
#19007=DIRECTION('ref_axis',(0.,0.,-1.));
#19008=DIRECTION('center_axis',(1.,0.,0.));
#19009=DIRECTION('ref_axis',(0.,0.,-1.));
#19010=DIRECTION('center_axis',(1.,0.,0.));
#19011=DIRECTION('ref_axis',(0.,0.,-1.));
#19012=DIRECTION('center_axis',(1.,0.,0.));
#19013=DIRECTION('ref_axis',(0.,0.,-1.));
#19014=DIRECTION('',(0.,0.,-1.));
#19015=DIRECTION('center_axis',(1.,0.,0.));
#19016=DIRECTION('ref_axis',(0.,0.,-1.));
#19017=DIRECTION('center_axis',(-1.,0.,0.));
#19018=DIRECTION('ref_axis',(0.,1.,0.));
#19019=DIRECTION('center_axis',(-1.,0.,0.));
#19020=DIRECTION('ref_axis',(0.,1.,0.));
#19021=DIRECTION('',(0.,0.,-1.));
#19022=DIRECTION('',(0.,1.,0.));
#19023=DIRECTION('',(0.,0.,-1.));
#19024=DIRECTION('center_axis',(0.,1.,0.));
#19025=DIRECTION('ref_axis',(1.,0.,0.));
#19026=DIRECTION('',(1.,0.,0.));
#19027=DIRECTION('',(1.,0.,0.));
#19028=DIRECTION('',(0.,0.,-1.));
#19029=DIRECTION('center_axis',(0.,-1.,0.));
#19030=DIRECTION('ref_axis',(-1.,0.,0.));
#19031=DIRECTION('',(-1.,0.,0.));
#19032=DIRECTION('',(0.,0.,-1.));
#19033=DIRECTION('',(-1.,0.,0.));
#19034=DIRECTION('center_axis',(1.,0.,0.));
#19035=DIRECTION('ref_axis',(0.,-1.,0.));
#19036=DIRECTION('center_axis',(1.,0.,0.));
#19037=DIRECTION('ref_axis',(0.,1.,0.));
#19038=DIRECTION('',(0.,-1.,0.));
#19039=DIRECTION('center_axis',(0.,0.,-1.));
#19040=DIRECTION('ref_axis',(-1.,0.,0.));
#19041=DIRECTION('center_axis',(0.,-0.88545602565321,0.464723172043769));
#19042=DIRECTION('ref_axis',(0.,-0.464723172043769,-0.88545602565321));
#19043=DIRECTION('center_axis',(1.,0.,0.));
#19044=DIRECTION('ref_axis',(0.,1.,0.));
#19045=DIRECTION('center_axis',(1.,0.,0.));
#19046=DIRECTION('ref_axis',(0.,1.,0.));
#19047=DIRECTION('center_axis',(1.,0.,0.));
#19048=DIRECTION('ref_axis',(0.,1.,0.));
#19049=DIRECTION('center_axis',(1.,0.,0.));
#19050=DIRECTION('ref_axis',(0.,1.,0.));
#19051=DIRECTION('center_axis',(1.,0.,0.));
#19052=DIRECTION('ref_axis',(0.,-0.239315664287557,0.970941817426052));
#19053=DIRECTION('center_axis',(1.,0.,0.));
#19054=DIRECTION('ref_axis',(0.,1.,0.));
#19055=DIRECTION('center_axis',(1.,0.,0.));
#19056=DIRECTION('ref_axis',(0.,1.,0.));
#19057=DIRECTION('center_axis',(1.,0.,0.));
#19058=DIRECTION('ref_axis',(0.,1.,0.));
#19059=DIRECTION('center_axis',(1.,0.,0.));
#19060=DIRECTION('ref_axis',(0.,1.,0.));
#19061=DIRECTION('center_axis',(1.,0.,0.));
#19062=DIRECTION('ref_axis',(0.,1.,0.));
#19063=DIRECTION('center_axis',(0.,-1.,0.));
#19064=DIRECTION('ref_axis',(0.,0.,-1.));
#19065=DIRECTION('center_axis',(1.,0.,0.));
#19066=DIRECTION('ref_axis',(0.,1.,0.));
#19067=DIRECTION('center_axis',(-1.,0.,0.));
#19068=DIRECTION('ref_axis',(0.,0.,1.));
#19069=DIRECTION('center_axis',(1.,0.,0.));
#19070=DIRECTION('ref_axis',(0.,0.,-1.));
#19071=DIRECTION('center_axis',(1.,0.,0.));
#19072=DIRECTION('ref_axis',(0.,1.,0.));
#19073=DIRECTION('center_axis',(1.,0.,0.));
#19074=DIRECTION('ref_axis',(0.,0.,-1.));
#19075=DIRECTION('',(-1.,0.,0.));
#19076=DIRECTION('center_axis',(1.,0.,0.));
#19077=DIRECTION('ref_axis',(0.,0.,-1.));
#19078=DIRECTION('center_axis',(1.,0.,0.));
#19079=DIRECTION('ref_axis',(0.,0.,-1.));
#19080=DIRECTION('center_axis',(1.,0.,0.));
#19081=DIRECTION('ref_axis',(0.,1.,0.));
#19082=DIRECTION('center_axis',(1.,0.,0.));
#19083=DIRECTION('ref_axis',(0.,0.,-1.));
#19084=DIRECTION('',(-1.,0.,0.));
#19085=DIRECTION('center_axis',(1.,0.,0.));
#19086=DIRECTION('ref_axis',(0.,0.,-1.));
#19087=DIRECTION('center_axis',(1.,0.,0.));
#19088=DIRECTION('ref_axis',(0.,0.,-1.));
#19089=DIRECTION('center_axis',(1.,0.,0.));
#19090=DIRECTION('ref_axis',(0.,1.,0.));
#19091=DIRECTION('center_axis',(1.,0.,0.));
#19092=DIRECTION('ref_axis',(0.,0.,-1.));
#19093=DIRECTION('',(-1.,0.,0.));
#19094=DIRECTION('center_axis',(-1.,0.,0.));
#19095=DIRECTION('ref_axis',(0.,1.,0.));
#19096=DIRECTION('center_axis',(1.,0.,0.));
#19097=DIRECTION('ref_axis',(0.,0.,-1.));
#19098=DIRECTION('',(-0.707106781186552,-0.707106781186543,-8.65956056235487E-17));
#19099=DIRECTION('center_axis',(1.,0.,0.));
#19100=DIRECTION('ref_axis',(0.,0.,-1.));
#25741=CARTESIAN_POINT('',(0.,0.,0.));
#25742=CARTESIAN_POINT('Origin',(-24.9,7.95870312499776,7.37391828833597));
#25743=CARTESIAN_POINT('',(-16.2963973586152,7.92227791262654,7.04797145648968));
#25744=CARTESIAN_POINT('',(-41.2927947172303,7.92227791262654,7.04797145648968));
#25745=CARTESIAN_POINT('',(-24.9,7.92227791262654,7.04797145648968));
#25746=CARTESIAN_POINT('',(-40.3,7.99512833736898,7.69986512018227));
#25747=CARTESIAN_POINT('Ctrl Pts',(-41.2927947172303,7.92227791262654,7.04797145648968));
#25748=CARTESIAN_POINT('Ctrl Pts',(-40.8162222946068,7.95787002002863,7.36646334414742));
#25749=CARTESIAN_POINT('Ctrl Pts',(-40.3,7.99512833736897,7.69986512018227));
#25750=CARTESIAN_POINT('',(-15.8,7.99512833736898,7.69986512018227));
#25751=CARTESIAN_POINT('',(-24.9,7.99512833736897,7.69986512018227));
#25752=CARTESIAN_POINT('Ctrl Pts',(-15.8,7.99512833736897,7.69986512018227));
#25753=CARTESIAN_POINT('Ctrl Pts',(-15.9670634484609,7.97101274591251,7.48406951813534));
#25754=CARTESIAN_POINT('Ctrl Pts',(-16.1329130514351,7.94669708059969,7.26648357815028));
#25755=CARTESIAN_POINT('Ctrl Pts',(-16.2963973586152,7.92227791262654,7.04797145648968));
#25756=CARTESIAN_POINT('Origin',(-24.9,9.71692839447408,4.8266892308878));
#25757=CARTESIAN_POINT('',(-15.8,10.0346105348206,4.74516505660943));
#25758=CARTESIAN_POINT('',(-40.3,10.0346105348206,4.74516505660943));
#25759=CARTESIAN_POINT('',(-24.9,10.0346105348206,4.74516505660943));
#25760=CARTESIAN_POINT('',(-41.2927947172303,9.39924625412754,4.90821340516617));
#25761=CARTESIAN_POINT('Ctrl Pts',(-40.3,10.0346105348206,4.74516505660943));
#25762=CARTESIAN_POINT('Ctrl Pts',(-40.816222294603,9.70966247747854,4.82855382385103));
#25763=CARTESIAN_POINT('Ctrl Pts',(-41.2927947172303,9.39924625412754,4.90821340516617));
#25764=CARTESIAN_POINT('',(-16.2963973586152,9.39924625412754,4.90821340516617));
#25765=CARTESIAN_POINT('',(-24.9,9.39924625412754,4.90821340516617));
#25766=CARTESIAN_POINT('Ctrl Pts',(-16.2963973586152,9.39924625412754,4.90821340516617));
#25767=CARTESIAN_POINT('Ctrl Pts',(-16.1329130514352,9.61221779340456,4.85356025763508));
#25768=CARTESIAN_POINT('Ctrl Pts',(-15.9670634484611,9.82428663522205,4.79913876198385));
#25769=CARTESIAN_POINT('Ctrl Pts',(-15.8,10.0346105348206,4.74516505660943));
#25770=CARTESIAN_POINT('Origin',(-16.05,0.,0.));
#25771=CARTESIAN_POINT('Origin',(-15.8,0.,0.));
#25772=CARTESIAN_POINT('',(-16.3,9.39625879385653,4.90615131023023));
#25773=CARTESIAN_POINT('Ctrl Pts',(-16.2963973586152,9.3992462541275,4.90821340516614));
#25774=CARTESIAN_POINT('Ctrl Pts',(-16.2981989900367,9.39775227019672,4.90718218251594));
#25775=CARTESIAN_POINT('Ctrl Pts',(-16.3,9.39625879385648,4.90615131023019));
#25776=CARTESIAN_POINT('',(-16.3,7.91929045235553,7.04590936155374));
#25777=CARTESIAN_POINT('Origin',(-16.3,0.,0.));
#25778=CARTESIAN_POINT('Ctrl Pts',(-16.3,7.91929045235555,7.04590936155372));
#25779=CARTESIAN_POINT('Ctrl Pts',(-16.2981989900367,7.92078392869578,7.04694023383947));
#25780=CARTESIAN_POINT('Ctrl Pts',(-16.2963973586152,7.92227791262655,7.04797145648966));
#25781=CARTESIAN_POINT('Origin',(-41.3,8.56123351384782,7.48901066372381));
#25782=CARTESIAN_POINT('',(-16.3,7.1621609418286,6.52330059428085));
#25783=CARTESIAN_POINT('',(-16.3,8.56123351384782,7.48901066372381));
#25784=CARTESIAN_POINT('',(-40.8,7.1621609418286,6.52330059428085));
#25785=CARTESIAN_POINT('',(-41.3,7.1621609418286,6.52330059428085));
#25786=CARTESIAN_POINT('',(-41.3,6.75066900888177,6.23926822091527));
#25787=CARTESIAN_POINT('',(-40.625,7.30618311835999,6.6227119249588));
#25788=CARTESIAN_POINT('',(-41.3,7.91929045235552,7.04590936155373));
#25789=CARTESIAN_POINT('',(-41.3,7.50107762221138,6.75723788780913));
#25790=CARTESIAN_POINT('Ctrl Pts',(-41.2927947172303,7.92227791262654,7.04797145648968));
#25791=CARTESIAN_POINT('Ctrl Pts',(-41.2963979800735,7.92078392869575,7.04694023383948));
#25792=CARTESIAN_POINT('Ctrl Pts',(-41.3,7.91929045235552,7.04590936155373));
#25793=CARTESIAN_POINT('Origin',(-16.3,8.60018139858871,5.93627660334058));
#25794=CARTESIAN_POINT('',(-16.3,8.63912928332961,4.38354254295734));
#25795=CARTESIAN_POINT('',(-16.3,8.63912928332961,4.38354254295734));
#25796=CARTESIAN_POINT('',(-16.3,7.1621609418286,6.52330059428085));
#25797=CARTESIAN_POINT('Origin',(-41.3,8.63912928332961,4.38354254295734));
#25798=CARTESIAN_POINT('',(-41.3,9.39625879385652,4.90615131023022));
#25799=CARTESIAN_POINT('Ctrl Pts',(-41.3,9.39625879385652,4.90615131023023));
#25800=CARTESIAN_POINT('Ctrl Pts',(-41.2963979800735,9.39775227019676,4.90718218251597));
#25801=CARTESIAN_POINT('Ctrl Pts',(-41.2927947172303,9.39924625412754,4.90821340516617));
#25802=CARTESIAN_POINT('',(-41.3,8.22763735038278,4.09951016959176));
#25803=CARTESIAN_POINT('',(-41.3,8.27850967770278,4.13462480176414));
#25804=CARTESIAN_POINT('',(-40.8,8.63912928332961,4.38354254295734));
#25805=CARTESIAN_POINT('',(-41.05,8.43338331685619,4.24152635627455));
#25806=CARTESIAN_POINT('',(-41.3,8.63912928332961,4.38354254295734));
#25807=CARTESIAN_POINT('Origin',(-24.9,10.4739123357613,2.83068661947788));
#25808=CARTESIAN_POINT('',(-16.2963973586152,10.2901843663683,2.55900267341252));
#25809=CARTESIAN_POINT('',(-41.2927947172303,10.2901843663683,2.55900267341252));
#25810=CARTESIAN_POINT('',(-24.9,10.2901843663683,2.55900267341252));
#25811=CARTESIAN_POINT('',(-40.3,10.6576403051544,3.10237056554323));
#25812=CARTESIAN_POINT('Ctrl Pts',(-41.2927947172303,10.2901843663683,2.55900267341252));
#25813=CARTESIAN_POINT('Ctrl Pts',(-40.8162222946067,10.4697101726358,2.82447275740919));
#25814=CARTESIAN_POINT('Ctrl Pts',(-40.3,10.6576403051544,3.10237056554323));
#25815=CARTESIAN_POINT('',(-15.8,10.6576403051544,3.10237056554323));
#25816=CARTESIAN_POINT('',(-24.9,10.6576403051544,3.10237056554323));
#25817=CARTESIAN_POINT('Ctrl Pts',(-15.8,10.6576403051544,3.10237056554324));
#25818=CARTESIAN_POINT('Ctrl Pts',(-15.9670634484609,10.5360017926907,2.92250012355864));
#25819=CARTESIAN_POINT('Ctrl Pts',(-16.1329130514351,10.4133541120997,2.741137395016));
#25820=CARTESIAN_POINT('Ctrl Pts',(-16.2963973586152,10.2901843663683,2.55900267341252));
#25821=CARTESIAN_POINT('Origin',(-24.9,10.8469871275755,-0.241860722557101));
#25822=CARTESIAN_POINT('',(-15.8,11.0903945201189,-0.461681045871784));
#25823=CARTESIAN_POINT('',(-40.3,11.0903945201189,-0.461681045871784));
#25824=CARTESIAN_POINT('',(-24.9,11.0903945201189,-0.461681045871784));
#25825=CARTESIAN_POINT('',(-41.2927947172303,10.6035797350322,-0.0220403992424186));
#25826=CARTESIAN_POINT('Ctrl Pts',(-40.3,11.0903945201189,-0.461681045871779));
#25827=CARTESIAN_POINT('Ctrl Pts',(-40.816222294603,10.8414199971464,-0.236833067488454));
#25828=CARTESIAN_POINT('Ctrl Pts',(-41.2927947172303,10.6035797350322,-0.0220403992424186));
#25829=CARTESIAN_POINT('',(-16.2963973586152,10.6035797350322,-0.0220403992424183));
#25830=CARTESIAN_POINT('',(-24.9,10.6035797350322,-0.0220403992424183));
#25831=CARTESIAN_POINT('Ctrl Pts',(-16.2963973586152,10.6035797350322,-0.022040399242419));
#25832=CARTESIAN_POINT('Ctrl Pts',(-16.1329130514351,10.7667580836949,-0.169406167332656));
#25833=CARTESIAN_POINT('Ctrl Pts',(-15.9670634484609,10.9292447874492,-0.316147313443247));
#25834=CARTESIAN_POINT('Ctrl Pts',(-15.8,11.0903945201189,-0.461681045871786));
#25835=CARTESIAN_POINT('Origin',(-16.05,0.,0.));
#25836=CARTESIAN_POINT('Origin',(-15.8,0.,0.));
#25837=CARTESIAN_POINT('',(-16.3,10.5999761670341,-0.022477951615418));
#25838=CARTESIAN_POINT('Ctrl Pts',(-16.2963973586153,10.6035797350322,-0.0220403992424162));
#25839=CARTESIAN_POINT('Ctrl Pts',(-16.2981989900368,10.6017776448974,-0.0222592126005309));
#25840=CARTESIAN_POINT('Ctrl Pts',(-16.3000000000001,10.5999761670342,-0.0224779516154164));
#25841=CARTESIAN_POINT('',(-16.3,10.2865807983703,2.55856512103952));
#25842=CARTESIAN_POINT('Origin',(-16.3,0.,0.));
#25843=CARTESIAN_POINT('Ctrl Pts',(-16.3000000000001,10.2865807983704,2.55856512103953));
#25844=CARTESIAN_POINT('Ctrl Pts',(-16.2981989900368,10.2883822762336,2.55878386005442));
#25845=CARTESIAN_POINT('Ctrl Pts',(-16.2963973586153,10.2901843663684,2.55900267341253));
#25846=CARTESIAN_POINT('Origin',(-41.3,11.0609125929761,2.65258602321261));
#25847=CARTESIAN_POINT('',(-16.3,9.3733075070094,2.44767366677856));
#25848=CARTESIAN_POINT('',(-16.3,11.0609125929761,2.65258602321261));
#25849=CARTESIAN_POINT('',(-40.8,9.3733075070094,2.44767366677856));
#25850=CARTESIAN_POINT('',(-41.3,9.3733075070094,2.44767366677856));
#25851=CARTESIAN_POINT('',(-41.3,8.87695306996037,2.3874053266509));
#25852=CARTESIAN_POINT('',(-40.625,9.54703155997656,2.46876758582325));
#25853=CARTESIAN_POINT('',(-41.3,10.2865807983703,2.55856512103952));
#25854=CARTESIAN_POINT('',(-41.3,10.6751032705011,2.60574029013207));
#25855=CARTESIAN_POINT('Ctrl Pts',(-41.2927947172303,10.2901843663683,2.55900267341252));
#25856=CARTESIAN_POINT('Ctrl Pts',(-41.2963979800735,10.2883822762335,2.5587838600544));
#25857=CARTESIAN_POINT('Ctrl Pts',(-41.3,10.2865807983703,2.55856512103952));
#25858=CARTESIAN_POINT('Origin',(-16.3,10.3738077343247,1.25960830866812));
#25859=CARTESIAN_POINT('',(-16.3,9.68670287567324,-0.133369405876376));
#25860=CARTESIAN_POINT('',(-16.3,9.68670287567324,-0.133369405876376));
#25861=CARTESIAN_POINT('',(-16.3,9.3733075070094,2.44767366677856));
#25862=CARTESIAN_POINT('Origin',(-41.3,9.68670287567324,-0.133369405876376));
#25863=CARTESIAN_POINT('',(-41.3,10.5999761670341,-0.0224779516154188));
#25864=CARTESIAN_POINT('Ctrl Pts',(-41.3,10.5999761670341,-0.0224779516154188));
#25865=CARTESIAN_POINT('Ctrl Pts',(-41.2963979800734,10.6017776448974,-0.022259212600532));
#25866=CARTESIAN_POINT('Ctrl Pts',(-41.2927947172303,10.6035797350322,-0.0220403992424185));
#25867=CARTESIAN_POINT('',(-41.3,9.19034843862421,-0.193637746004037));
#25868=CARTESIAN_POINT('',(-41.3,10.1446960961816,-0.0777589607398988));
#25869=CARTESIAN_POINT('',(-40.8,9.68670287567324,-0.133369405876376));
#25870=CARTESIAN_POINT('',(-41.05,9.43852565714873,-0.163503575940206));
#25871=CARTESIAN_POINT('',(-41.3,9.68670287567324,-0.133369405876376));
#25872=CARTESIAN_POINT('Origin',(-24.9,10.589674454729,-2.36102124043076));
#25873=CARTESIAN_POINT('',(-16.2963973586152,10.30073359194,-2.51620278281809));
#25874=CARTESIAN_POINT('',(-41.2927947172303,10.30073359194,-2.51620278281809));
#25875=CARTESIAN_POINT('',(-24.9,10.30073359194,-2.51620278281809));
#25876=CARTESIAN_POINT('',(-40.3,10.8786153175179,-2.20583969804344));
#25877=CARTESIAN_POINT('Ctrl Pts',(-41.2927947172303,10.30073359194,-2.51620278281809));
#25878=CARTESIAN_POINT('Ctrl Pts',(-40.8162222946069,10.5830658983774,-2.36457049946494));
#25879=CARTESIAN_POINT('Ctrl Pts',(-40.3,10.8786153175179,-2.20583969804344));
#25880=CARTESIAN_POINT('',(-15.8,10.8786153175179,-2.20583969804344));
#25881=CARTESIAN_POINT('',(-24.9,10.8786153175179,-2.20583969804344));
#25882=CARTESIAN_POINT('Ctrl Pts',(-15.8,10.8786153175179,-2.20583969804343));
#25883=CARTESIAN_POINT('Ctrl Pts',(-15.967063448461,10.6873198013494,-2.30857882938082));
#25884=CARTESIAN_POINT('Ctrl Pts',(-16.1329130514351,10.4944372110389,-2.41217033102974));
#25885=CARTESIAN_POINT('Ctrl Pts',(-16.2963973586152,10.30073359194,-2.51620278281809));
#25886=CARTESIAN_POINT('Origin',(-24.9,9.49213183011501,-5.25500329920184));
#25887=CARTESIAN_POINT('',(-15.8,9.60550277460058,-5.56276158460351));
#25888=CARTESIAN_POINT('',(-40.3,9.60550277460058,-5.56276158460351));
#25889=CARTESIAN_POINT('',(-24.9,9.60550277460058,-5.56276158460351));
#25890=CARTESIAN_POINT('',(-41.2927947172303,9.37876088562945,-4.94724501380017));
#25891=CARTESIAN_POINT('Ctrl Pts',(-40.3,9.60550277460057,-5.56276158460351));
#25892=CARTESIAN_POINT('Ctrl Pts',(-40.8162222946031,9.48953884874235,-5.24796435721412));
#25893=CARTESIAN_POINT('Ctrl Pts',(-41.2927947172303,9.37876088562945,-4.94724501380017));
#25894=CARTESIAN_POINT('',(-16.2963973586152,9.37876088562945,-4.94724501380017));
#25895=CARTESIAN_POINT('',(-24.9,9.37876088562945,-4.94724501380017));
#25896=CARTESIAN_POINT('Ctrl Pts',(-16.2963973586152,9.37876088562945,-4.94724501380017));
#25897=CARTESIAN_POINT('Ctrl Pts',(-16.1329130514351,9.45476385051142,-5.15356368093007));
#25898=CARTESIAN_POINT('Ctrl Pts',(-15.9670634484609,9.53044467054932,-5.35900784934856));
#25899=CARTESIAN_POINT('Ctrl Pts',(-15.8,9.60550277460058,-5.56276158460352));
#25900=CARTESIAN_POINT('Origin',(-16.05,0.,0.));
#25901=CARTESIAN_POINT('Origin',(-15.8,0.,0.));
#25902=CARTESIAN_POINT('',(-16.3,9.37536674390501,-4.94595778563465));
#25903=CARTESIAN_POINT('Ctrl Pts',(-16.2963973586152,9.37876088562946,-4.94724501380016));
#25904=CARTESIAN_POINT('Ctrl Pts',(-16.2981989900368,9.37706352642295,-4.94660129036284));
#25905=CARTESIAN_POINT('Ctrl Pts',(-16.3000000000001,9.37536674390502,-4.94595778563464));
#25906=CARTESIAN_POINT('',(-16.3,10.2973394502156,-2.51491555465257));
#25907=CARTESIAN_POINT('Origin',(-16.3,0.,0.));
#25908=CARTESIAN_POINT('Ctrl Pts',(-16.3,10.2973394502156,-2.51491555465259));
#25909=CARTESIAN_POINT('Ctrl Pts',(-16.2981989900368,10.2990362327336,-2.51555905938079));
#25910=CARTESIAN_POINT('Ctrl Pts',(-16.2963973586152,10.3007335919401,-2.51620278281811));
#25911=CARTESIAN_POINT('Origin',(-41.3,11.0266698955005,-2.79151410808962));
#25912=CARTESIAN_POINT('',(-16.3,9.43714228293528,-2.18868580011731));
#25913=CARTESIAN_POINT('',(-16.3,11.0266698955005,-2.79151410808962));
#25914=CARTESIAN_POINT('',(-40.8,9.43714228293528,-2.18868580011731));
#25915=CARTESIAN_POINT('',(-41.3,9.43714228293528,-2.18868580011731));
#25916=CARTESIAN_POINT('',(-41.3,8.96963416159257,-2.01138335659604));
#25917=CARTESIAN_POINT('',(-40.625,9.60077012540523,-2.25074165534975));
#25918=CARTESIAN_POINT('',(-41.3,10.2973394502156,-2.51491555465257));
#25919=CARTESIAN_POINT('',(-41.3,10.3773816069813,-2.5452715406374));
#25920=CARTESIAN_POINT('Ctrl Pts',(-41.2927947172303,10.30073359194,-2.51620278281809));
#25921=CARTESIAN_POINT('Ctrl Pts',(-41.2963979800735,10.2990362327335,-2.51555905938076));
#25922=CARTESIAN_POINT('Ctrl Pts',(-41.3,10.2973394502156,-2.51491555465257));
#25923=CARTESIAN_POINT('Origin',(-16.3,9.77091973606258,-3.7056210695945));
#25924=CARTESIAN_POINT('',(-16.3,8.51516957662468,-4.61972803109938));
#25925=CARTESIAN_POINT('',(-16.3,8.51516957662468,-4.61972803109938));
#25926=CARTESIAN_POINT('',(-16.3,9.43714228293528,-2.18868580011731));
#25927=CARTESIAN_POINT('Origin',(-41.3,8.51516957662468,-4.61972803109938));
#25928=CARTESIAN_POINT('',(-41.3,9.375366743905,-4.94595778563465));
#25929=CARTESIAN_POINT('Ctrl Pts',(-41.3,9.375366743905,-4.94595778563465));
#25930=CARTESIAN_POINT('Ctrl Pts',(-41.2963979800735,9.37706352642292,-4.94660129036284));
#25931=CARTESIAN_POINT('Ctrl Pts',(-41.2927947172303,9.37876088562945,-4.94724501380017));
#25932=CARTESIAN_POINT('',(-41.3,8.04766145528198,-4.44242558757812));
#25933=CARTESIAN_POINT('',(-41.3,8.66064509438811,-4.67489961763332));
#25934=CARTESIAN_POINT('',(-40.8,8.51516957662468,-4.61972803109938));
#25935=CARTESIAN_POINT('',(-41.05,8.28141551595333,-4.53107680933875));
#25936=CARTESIAN_POINT('',(-41.3,8.51516957662468,-4.61972803109938));
#25937=CARTESIAN_POINT('Origin',(-24.9,8.27946977552995,-7.01184758754715));
#25938=CARTESIAN_POINT('',(-16.2963973586152,7.95150888889516,-7.01497650503583));
#25939=CARTESIAN_POINT('',(-41.2927947172303,7.95150888889516,-7.01497650503583));
#25940=CARTESIAN_POINT('',(-24.9,7.95150888889516,-7.01497650503583));
#25941=CARTESIAN_POINT('',(-40.3,8.60743066216474,-7.00871867005848));
#25942=CARTESIAN_POINT('Ctrl Pts',(-41.2927947172303,7.95150888889516,-7.01497650503583));
#25943=CARTESIAN_POINT('Ctrl Pts',(-40.816222294607,8.2719687665707,-7.01191915107522));
#25944=CARTESIAN_POINT('Ctrl Pts',(-40.3,8.60743066216473,-7.00871867005847));
#25945=CARTESIAN_POINT('',(-15.8,8.60743066216474,-7.00871867005848));
#25946=CARTESIAN_POINT('',(-24.9,8.60743066216474,-7.00871867005848));
#25947=CARTESIAN_POINT('Ctrl Pts',(-15.8,8.60743066216474,-7.00871867005848));
#25948=CARTESIAN_POINT('Ctrl Pts',(-15.967063448461,8.39030163968471,-7.01079019389995));
#25949=CARTESIAN_POINT('Ctrl Pts',(-16.1329130514352,8.17137121660765,-7.01287890404036));
#25950=CARTESIAN_POINT('Ctrl Pts',(-16.2963973586152,7.95150888889516,-7.01497650503583));
#25951=CARTESIAN_POINT('Origin',(-24.9,5.96274352296442,-9.06428794965444));
#25952=CARTESIAN_POINT('',(-15.8,5.92010610227854,-9.38948048284698));
#25953=CARTESIAN_POINT('',(-40.3,5.92010610227854,-9.38948048284698));
#25954=CARTESIAN_POINT('',(-24.9,5.92010610227854,-9.38948048284698));
#25955=CARTESIAN_POINT('',(-41.2927947172303,6.0053809436503,-8.7390954164619));
#25956=CARTESIAN_POINT('Ctrl Pts',(-40.3,5.92010610227854,-9.38948048284697));
#25957=CARTESIAN_POINT('Ctrl Pts',(-40.8162222946032,5.96371871143196,-9.05685025752861));
#25958=CARTESIAN_POINT('Ctrl Pts',(-41.2927947172303,6.0053809436503,-8.7390954164619));
#25959=CARTESIAN_POINT('',(-16.2963973586152,6.0053809436503,-8.7390954164619));
#25960=CARTESIAN_POINT('',(-24.9,6.0053809436503,-8.7390954164619));
#25961=CARTESIAN_POINT('Ctrl Pts',(-16.2963973586152,6.0053809436503,-8.73909541646189));
#25962=CARTESIAN_POINT('Ctrl Pts',(-16.1329130514351,5.97679716143209,-8.95710186240153));
#25963=CARTESIAN_POINT('Ctrl Pts',(-15.9670634484609,5.94833453393568,-9.17418427001393));
#25964=CARTESIAN_POINT('Ctrl Pts',(-15.8,5.92010610227854,-9.38948048284698));
#25965=CARTESIAN_POINT('Origin',(-16.05,0.,0.));
#25966=CARTESIAN_POINT('Origin',(-15.8,0.,0.));
#25967=CARTESIAN_POINT('',(-16.3,6.0029737851647,-8.7363782962178));
#25968=CARTESIAN_POINT('Ctrl Pts',(-16.2963973586153,6.00538094365033,-8.73909541646192));
#25969=CARTESIAN_POINT('Ctrl Pts',(-16.2981989900368,6.00417715991094,-8.73773662551094));
#25970=CARTESIAN_POINT('Ctrl Pts',(-16.3000000000001,6.00297378516472,-8.73637829621782));
#25971=CARTESIAN_POINT('',(-16.3,7.94910173040956,-7.01225938479173));
#25972=CARTESIAN_POINT('Origin',(-16.3,0.,0.));
#25973=CARTESIAN_POINT('Ctrl Pts',(-16.3000000000001,7.94910173040962,-7.01225938479175));
#25974=CARTESIAN_POINT('Ctrl Pts',(-16.2981989900368,7.95030510515584,-7.01361771408487));
#25975=CARTESIAN_POINT('Ctrl Pts',(-16.2963973586152,7.95150888889523,-7.01497650503585));
#25976=CARTESIAN_POINT('Origin',(-41.3,8.46635001074342,-7.59611199862041));
#25977=CARTESIAN_POINT('',(-16.3,7.33904149173406,-6.32364372672954));
#25978=CARTESIAN_POINT('',(-16.3,8.46635001074342,-7.59611199862041));
#25979=CARTESIAN_POINT('',(-40.8,7.33904149173406,-6.32364372672954));
#25980=CARTESIAN_POINT('',(-41.3,7.33904149173406,-6.32364372672954));
#25981=CARTESIAN_POINT('',(-41.3,7.00748016261367,-5.94938835264399));
#25982=CARTESIAN_POINT('',(-40.625,7.4550879569262,-6.45463310765948));
#25983=CARTESIAN_POINT('',(-41.3,7.94910173040956,-7.01225938479173));
#25984=CARTESIAN_POINT('',(-41.3,7.05028478900632,-5.99770478781353));
#25985=CARTESIAN_POINT('Ctrl Pts',(-41.2927947172303,7.95150888889516,-7.01497650503583));
#25986=CARTESIAN_POINT('Ctrl Pts',(-41.2963979800735,7.95030510515576,-7.01361771408484));
#25987=CARTESIAN_POINT('Ctrl Pts',(-41.3,7.94910173040956,-7.01225938479173));
#25988=CARTESIAN_POINT('Origin',(-16.3,6.92963177861631,-7.82193731838801));
#25989=CARTESIAN_POINT('',(-16.3,5.3929135464892,-8.04776263815561));
#25990=CARTESIAN_POINT('',(-16.3,5.3929135464892,-8.04776263815561));
#25991=CARTESIAN_POINT('',(-16.3,7.33904149173406,-6.32364372672954));
#25992=CARTESIAN_POINT('Origin',(-41.3,5.3929135464892,-8.04776263815561));
#25993=CARTESIAN_POINT('',(-41.3,6.00297378516469,-8.7363782962178));
#25994=CARTESIAN_POINT('Ctrl Pts',(-41.3,6.00297378516469,-8.7363782962178));
#25995=CARTESIAN_POINT('Ctrl Pts',(-41.2963979800734,6.00417715991092,-8.73773662551093));
#25996=CARTESIAN_POINT('Ctrl Pts',(-41.2927947172303,6.0053809436503,-8.7390954164619));
#25997=CARTESIAN_POINT('',(-41.3,5.0613522173688,-7.67350726407006));
#25998=CARTESIAN_POINT('',(-41.3,4.54050258425678,-7.08558956329416));
#25999=CARTESIAN_POINT('',(-40.8,5.3929135464892,-8.04776263815561));
#26000=CARTESIAN_POINT('',(-41.05,5.227132881929,-7.86063495111283));
#26001=CARTESIAN_POINT('',(-41.3,5.3929135464892,-8.04776263815561));
#26002=CARTESIAN_POINT('Origin',(-24.9,4.07253834918427,-10.0563441542803));
#26003=CARTESIAN_POINT('',(-41.2927947172303,3.78068932547452,-9.90670364958125));
#26004=CARTESIAN_POINT('',(-40.3,4.36438737289401,-10.2059846589794));
#26005=CARTESIAN_POINT('Ctrl Pts',(-41.2927947172303,3.78068932547452,-9.90670364958125));
#26006=CARTESIAN_POINT('Ctrl Pts',(-40.8162222946071,4.06586327837296,-10.0529216279604));
#26007=CARTESIAN_POINT('Ctrl Pts',(-40.3,4.364387372894,-10.2059846589794));
#26008=CARTESIAN_POINT('',(-15.8,4.36438737289401,-10.2059846589794));
#26009=CARTESIAN_POINT('',(-24.9,4.36438737289401,-10.2059846589794));
#26010=CARTESIAN_POINT('',(-16.2963973586152,3.78068932547452,-9.90670364958125));
#26011=CARTESIAN_POINT('Ctrl Pts',(-16.2963973586435,3.78068932544062,-9.90670364956387));
#26012=CARTESIAN_POINT('Ctrl Pts',(-16.0581111473186,4.06586327835559,-10.0529216279515));
#26013=CARTESIAN_POINT('Ctrl Pts',(-15.8,4.36438737289401,-10.2059846589794));
#26014=CARTESIAN_POINT('',(-24.9,3.78068932547452,-9.90670364958125));
#26015=CARTESIAN_POINT('Origin',(-41.3,3.96649136910327,-10.6605321733406));
#26016=CARTESIAN_POINT('',(-16.3,3.7798206012274,-9.90317909676165));
#26017=CARTESIAN_POINT('Ctrl Pts',(-16.2963973586156,3.78068932547441,-9.90670364958079));
#26018=CARTESIAN_POINT('Ctrl Pts',(-16.2981989900369,3.78025488954973,-9.90494107374806));
#26019=CARTESIAN_POINT('Ctrl Pts',(-16.3,3.7798206012274,-9.90317909676165));
#26020=CARTESIAN_POINT('',(-16.3,3.55965473981442,-9.00993108371628));
#26021=CARTESIAN_POINT('',(-16.3,3.96649136910327,-10.6605321733406));
#26022=CARTESIAN_POINT('',(-40.8,3.55965473981442,-9.00993108371628));
#26023=CARTESIAN_POINT('',(-41.3,3.55965473981442,-9.00993108371628));
#26024=CARTESIAN_POINT('',(-41.3,3.43999690767064,-8.52446017500325));
#26025=CARTESIAN_POINT('',(-40.625,3.60153498106474,-9.17984590176584));
#26026=CARTESIAN_POINT('',(-41.3,3.7798206012274,-9.90317909676164));
#26027=CARTESIAN_POINT('',(-41.3,2.91789939789756,-6.40622731079936));
#26028=CARTESIAN_POINT('Ctrl Pts',(-41.2927947172303,3.78068932547452,-9.90670364958125));
#26029=CARTESIAN_POINT('Ctrl Pts',(-41.2963979800735,3.78025488954977,-9.90494107374824));
#26030=CARTESIAN_POINT('Ctrl Pts',(-41.3,3.7798206012274,-9.90317909676164));
#26031=CARTESIAN_POINT('Origin',(-24.9,1.06736253355198,-10.7970534673528));
#26032=CARTESIAN_POINT('',(-15.8,0.878484466937167,-11.0651825579766));
#26033=CARTESIAN_POINT('',(-40.3,0.878484466937167,-11.0651825579766));
#26034=CARTESIAN_POINT('',(-24.9,0.878484466937167,-11.0651825579766));
#26035=CARTESIAN_POINT('',(-41.2927947172303,1.25624060016678,-10.5289243767289));
#26036=CARTESIAN_POINT('Ctrl Pts',(-40.3,0.878484466937173,-11.0651825579766));
#26037=CARTESIAN_POINT('Ctrl Pts',(-40.816222294603,1.07168248793402,-10.7909209107211));
#26038=CARTESIAN_POINT('Ctrl Pts',(-41.2927947172303,1.25624060016679,-10.5289243767289));
#26039=CARTESIAN_POINT('',(-16.2963973586152,1.25624060016678,-10.5289243767289));
#26040=CARTESIAN_POINT('',(-24.9,1.25624060016678,-10.5289243767289));
#26041=CARTESIAN_POINT('Ctrl Pts',(-16.2963973586152,1.25624060016679,-10.5289243767289));
#26042=CARTESIAN_POINT('Ctrl Pts',(-16.1329130514352,1.12961827088273,-10.7086759519758));
#26043=CARTESIAN_POINT('Ctrl Pts',(-15.9670634484611,1.00353264079967,-10.8876656353246));
#26044=CARTESIAN_POINT('Ctrl Pts',(-15.8,0.878484466937165,-11.0651825579766));
#26045=CARTESIAN_POINT('Origin',(-16.05,0.,0.));
#26046=CARTESIAN_POINT('',(-16.3,1.25537187591967,-10.5253998239093));
#26047=CARTESIAN_POINT('Origin',(-16.3,0.,0.));
#26048=CARTESIAN_POINT('Origin',(-15.8,0.,0.));
#26049=CARTESIAN_POINT('Ctrl Pts',(-16.2963973586152,1.25624060016679,-10.5289243767289));
#26050=CARTESIAN_POINT('Ctrl Pts',(-16.2981989900367,1.25580616424205,-10.5271618008959));
#26051=CARTESIAN_POINT('Ctrl Pts',(-16.3,1.25537187591967,-10.5253998239093));
#26052=CARTESIAN_POINT('Origin',(-41.3,1.03520601450668,-9.63215181086392));
#26053=CARTESIAN_POINT('',(-41.3,1.25537187591967,-10.5253998239093));
#26054=CARTESIAN_POINT('Ctrl Pts',(-41.3,1.25537187591967,-10.5253998239093));
#26055=CARTESIAN_POINT('Ctrl Pts',(-41.2963979800735,1.25580616424204,-10.5271618008959));
#26056=CARTESIAN_POINT('Ctrl Pts',(-41.2927947172303,1.25624060016679,-10.5289243767289));
#26057=CARTESIAN_POINT('',(-41.3,0.915548182362905,-9.1466809021509));
#26058=CARTESIAN_POINT('',(-41.3,0.1900323579454,-6.20314749313486));
#26059=CARTESIAN_POINT('',(-40.8,1.03520601450668,-9.63215181086392));
#26060=CARTESIAN_POINT('',(-41.05,0.975377098434795,-9.38941635650741));
#26061=CARTESIAN_POINT('',(-16.3,1.03520601450668,-9.63215181086392));
#26062=CARTESIAN_POINT('',(-41.3,1.03520601450668,-9.63215181086392));
#26063=CARTESIAN_POINT('',(-16.3,1.03520601450668,-9.63215181086392));
#26064=CARTESIAN_POINT('Origin',(-40.8,0.,0.));
#26065=CARTESIAN_POINT('',(-40.3,-0.878484466937175,-11.0651825579766));
#26066=CARTESIAN_POINT('Origin',(-40.3,0.,0.));
#26067=CARTESIAN_POINT('',(-41.2927947172303,-1.25624060016679,-10.5289243767289));
#26068=CARTESIAN_POINT('Ctrl Pts',(-41.2927947172303,-1.25624060016679,
-10.5289243767289));
#26069=CARTESIAN_POINT('Ctrl Pts',(-40.8162222946063,-1.07168248793539,
-10.7909209107192));
#26070=CARTESIAN_POINT('Ctrl Pts',(-40.3,-0.878484466937179,-11.0651825579766));
#26071=CARTESIAN_POINT('',(-41.3,-1.25537187591967,-10.5253998239093));
#26072=CARTESIAN_POINT('Ctrl Pts',(-41.2927947172303,-1.25624060016679,
-10.5289243767289));
#26073=CARTESIAN_POINT('Ctrl Pts',(-41.2963979800735,-1.25580616424205,
-10.5271618008959));
#26074=CARTESIAN_POINT('Ctrl Pts',(-41.3,-1.25537187591967,-10.5253998239093));
#26075=CARTESIAN_POINT('Origin',(-41.3,0.,0.));
#26076=CARTESIAN_POINT('Origin',(-24.9,0.,0.));
#26077=CARTESIAN_POINT('',(-9.49999999999999,-11.1,-1.35935794705356E-15));
#26078=CARTESIAN_POINT('Origin',(-9.49999999999999,0.,0.));
#26079=CARTESIAN_POINT('',(-15.8,-11.1,-1.35935794705356E-15));
#26080=CARTESIAN_POINT('',(-24.9,-11.1,-1.35935794705356E-15));
#26081=CARTESIAN_POINT('',(-15.8,-11.0903945201189,-0.461681045871775));
#26082=CARTESIAN_POINT('Origin',(-15.8,0.,0.));
#26083=CARTESIAN_POINT('',(-40.3,-11.0903945201189,-0.461681045871775));
#26084=CARTESIAN_POINT('',(-24.9,-11.0903945201189,-0.461681045871775));
#26085=CARTESIAN_POINT('',(-40.3,-10.8786153175179,-2.20583969804343));
#26086=CARTESIAN_POINT('Origin',(-40.3,0.,0.));
#26087=CARTESIAN_POINT('',(-15.8,-10.8786153175179,-2.20583969804343));
#26088=CARTESIAN_POINT('',(-24.9,-10.8786153175179,-2.20583969804343));
#26089=CARTESIAN_POINT('',(-15.8,-9.60550277460058,-5.56276158460351));
#26090=CARTESIAN_POINT('Origin',(-15.8,0.,0.));
#26091=CARTESIAN_POINT('',(-40.3,-9.60550277460058,-5.56276158460351));
#26092=CARTESIAN_POINT('',(-24.9,-9.60550277460058,-5.56276158460351));
#26093=CARTESIAN_POINT('',(-40.3,-8.60743066216474,-7.00871867005847));
#26094=CARTESIAN_POINT('Origin',(-40.3,0.,0.));
#26095=CARTESIAN_POINT('',(-15.8,-8.60743066216474,-7.00871867005847));
#26096=CARTESIAN_POINT('',(-24.9,-8.60743066216474,-7.00871867005847));
#26097=CARTESIAN_POINT('',(-15.8,-5.92010610227855,-9.38948048284698));
#26098=CARTESIAN_POINT('Origin',(-15.8,0.,0.));
#26099=CARTESIAN_POINT('',(-40.3,-5.92010610227855,-9.38948048284698));
#26100=CARTESIAN_POINT('',(-24.9,-5.92010610227855,-9.38948048284698));
#26101=CARTESIAN_POINT('',(-40.3,-4.36438737289401,-10.2059846589794));
#26102=CARTESIAN_POINT('Origin',(-40.3,0.,0.));
#26103=CARTESIAN_POINT('',(-15.8,-4.36438737289401,-10.2059846589794));
#26104=CARTESIAN_POINT('',(-24.9,-4.36438737289401,-10.2059846589794));
#26105=CARTESIAN_POINT('',(-15.8,-0.878484466937174,-11.0651825579766));
#26106=CARTESIAN_POINT('Origin',(-15.8,0.,0.));
#26107=CARTESIAN_POINT('',(-24.9,-0.878484466937175,-11.0651825579766));
#26108=CARTESIAN_POINT('Origin',(-40.3,0.,0.));
#26109=CARTESIAN_POINT('Origin',(-40.3,0.,0.));
#26110=CARTESIAN_POINT('Origin',(-40.3,0.,0.));
#26111=CARTESIAN_POINT('Origin',(-40.3,0.,0.));
#26112=CARTESIAN_POINT('',(-40.3,6.68001820616131,8.86495103005952));
#26113=CARTESIAN_POINT('Origin',(-40.3,0.,0.));
#26114=CARTESIAN_POINT('',(-15.8,6.68001820616131,8.86495103005952));
#26115=CARTESIAN_POINT('',(-24.9,6.68001820616131,8.86495103005952));
#26116=CARTESIAN_POINT('',(-15.8,3.50102881923381,10.5334133692215));
#26117=CARTESIAN_POINT('Origin',(-15.8,0.,0.));
#26118=CARTESIAN_POINT('',(-40.3,3.50102881923381,10.5334133692215));
#26119=CARTESIAN_POINT('',(-24.9,3.50102881923381,10.5334133692215));
#26120=CARTESIAN_POINT('',(-40.3,1.79511420941674,10.9538835567642));
#26121=CARTESIAN_POINT('Origin',(-40.3,0.,0.));
#26122=CARTESIAN_POINT('',(-15.8,1.79511420941674,10.9538835567642));
#26123=CARTESIAN_POINT('',(-24.9,1.79511420941674,10.9538835567642));
#26124=CARTESIAN_POINT('',(-15.8,-1.79511420941674,10.9538835567642));
#26125=CARTESIAN_POINT('Origin',(-15.8,0.,0.));
#26126=CARTESIAN_POINT('',(-40.3,-1.79511420941674,10.9538835567642));
#26127=CARTESIAN_POINT('',(-24.9,-1.79511420941674,10.9538835567642));
#26128=CARTESIAN_POINT('',(-40.3,-3.50102881923381,10.5334133692215));
#26129=CARTESIAN_POINT('Origin',(-40.3,0.,0.));
#26130=CARTESIAN_POINT('',(-15.8,-3.50102881923381,10.5334133692215));
#26131=CARTESIAN_POINT('',(-24.9,-3.50102881923381,10.5334133692215));
#26132=CARTESIAN_POINT('',(-15.8,-6.68001820616131,8.86495103005953));
#26133=CARTESIAN_POINT('Origin',(-15.8,0.,0.));
#26134=CARTESIAN_POINT('',(-40.3,-6.68001820616131,8.86495103005953));
#26135=CARTESIAN_POINT('',(-24.9,-6.68001820616131,8.86495103005953));
#26136=CARTESIAN_POINT('',(-40.3,-7.99512833736897,7.69986512018227));
#26137=CARTESIAN_POINT('Origin',(-40.3,0.,0.));
#26138=CARTESIAN_POINT('',(-15.8,-7.99512833736897,7.69986512018227));
#26139=CARTESIAN_POINT('',(-24.9,-7.99512833736897,7.69986512018227));
#26140=CARTESIAN_POINT('',(-15.8,-10.0346105348206,4.74516505660943));
#26141=CARTESIAN_POINT('Origin',(-15.8,0.,0.));
#26142=CARTESIAN_POINT('',(-40.3,-10.0346105348206,4.74516505660943));
#26143=CARTESIAN_POINT('',(-24.9,-10.0346105348206,4.74516505660943));
#26144=CARTESIAN_POINT('',(-40.3,-10.6576403051544,3.10237056554324));
#26145=CARTESIAN_POINT('Origin',(-40.3,0.,0.));
#26146=CARTESIAN_POINT('',(-15.8,-10.6576403051544,3.10237056554324));
#26147=CARTESIAN_POINT('',(-24.9,-10.6576403051544,3.10237056554324));
#26148=CARTESIAN_POINT('Origin',(-15.8,0.,0.));
#26149=CARTESIAN_POINT('Origin',(-24.9,-1.06736253355198,-10.7970534673528));
#26150=CARTESIAN_POINT('',(-16.2963973586152,-1.25624060016679,-10.5289243767289));
#26151=CARTESIAN_POINT('',(-24.9,-1.25624060016679,-10.5289243767289));
#26152=CARTESIAN_POINT('Ctrl Pts',(-15.8,-0.878484466937174,-11.0651825579766));
#26153=CARTESIAN_POINT('Ctrl Pts',(-15.967063448461,-1.00353264079959,-10.8876656353247));
#26154=CARTESIAN_POINT('Ctrl Pts',(-16.1329130514351,-1.1296182708827,-10.7086759519759));
#26155=CARTESIAN_POINT('Ctrl Pts',(-16.2963973586152,-1.25624060016679,
-10.5289243767289));
#26156=CARTESIAN_POINT('Origin',(-24.9,-4.07253834918427,-10.0563441542803));
#26157=CARTESIAN_POINT('',(-41.2927947172303,-3.78068932547453,-9.90670364958125));
#26158=CARTESIAN_POINT('Ctrl Pts',(-40.3,-4.36438737289401,-10.2059846589794));
#26159=CARTESIAN_POINT('Ctrl Pts',(-40.8162222946027,-4.06586327837569,
-10.0529216279618));
#26160=CARTESIAN_POINT('Ctrl Pts',(-41.2927947172303,-3.78068932547453,
-9.90670364958125));
#26161=CARTESIAN_POINT('',(-16.2963973586152,-3.78068932547453,-9.90670364958125));
#26162=CARTESIAN_POINT('',(-24.9,-3.78068932547453,-9.90670364958125));
#26163=CARTESIAN_POINT('Ctrl Pts',(-16.2963973586152,-3.78068932547453,
-9.90670364958125));
#26164=CARTESIAN_POINT('Ctrl Pts',(-16.1329130514351,-3.97634255215008,
-10.0070214344879));
#26165=CARTESIAN_POINT('Ctrl Pts',(-15.9670634484608,-4.17116648646451,
-10.1069140141776));
#26166=CARTESIAN_POINT('Ctrl Pts',(-15.8,-4.36438737289401,-10.2059846589794));
#26167=CARTESIAN_POINT('Origin',(-16.05,0.,0.));
#26168=CARTESIAN_POINT('',(-16.3,-3.77982060122741,-9.90317909676165));
#26169=CARTESIAN_POINT('Ctrl Pts',(-16.2963973586152,-3.78068932547454,
-9.9067036495813));
#26170=CARTESIAN_POINT('Ctrl Pts',(-16.2981989900368,-3.7802548895498,-9.90494107374833));
#26171=CARTESIAN_POINT('Ctrl Pts',(-16.3000000000001,-3.77982060122742,
-9.9031790967617));
#26172=CARTESIAN_POINT('',(-16.3,-1.25537187591967,-10.5253998239093));
#26173=CARTESIAN_POINT('Origin',(-16.3,0.,0.));
#26174=CARTESIAN_POINT('Ctrl Pts',(-16.3,-1.25537187591968,-10.5253998239093));
#26175=CARTESIAN_POINT('Ctrl Pts',(-16.2981989900368,-1.25580616424205,
-10.527161800896));
#26176=CARTESIAN_POINT('Ctrl Pts',(-16.2963973586152,-1.25624060016679,
-10.5289243767289));
#26177=CARTESIAN_POINT('Origin',(-41.3,-1.44204264379554,-11.2827529004882));
#26178=CARTESIAN_POINT('',(-16.3,-1.03520601450669,-9.63215181086392));
#26179=CARTESIAN_POINT('',(-16.3,-1.44204264379554,-11.2827529004882));
#26180=CARTESIAN_POINT('',(-40.8,-1.03520601450669,-9.63215181086392));
#26181=CARTESIAN_POINT('',(-41.3,-1.03520601450669,-9.63215181086392));
#26182=CARTESIAN_POINT('',(-41.3,-0.915548182362911,-9.1466809021509));
#26183=CARTESIAN_POINT('',(-40.625,-1.07708625575701,-9.80206662891349));
#26184=CARTESIAN_POINT('',(-41.3,0.213632391448158,-4.56541522611503));
#26185=CARTESIAN_POINT('Origin',(-16.3,-2.50084869180498,-10.1463419921022));
#26186=CARTESIAN_POINT('',(-16.3,-3.55965473981442,-9.00993108371627));
#26187=CARTESIAN_POINT('',(-16.3,-3.55965473981442,-9.00993108371627));
#26188=CARTESIAN_POINT('',(-16.3,-1.03520601450669,-9.63215181086392));
#26189=CARTESIAN_POINT('Origin',(-41.3,-3.55965473981442,-9.00993108371627));
#26190=CARTESIAN_POINT('',(-41.3,-3.77982060122741,-9.90317909676164));
#26191=CARTESIAN_POINT('Ctrl Pts',(-41.3,-3.77982060122741,-9.90317909676164));
#26192=CARTESIAN_POINT('Ctrl Pts',(-41.2963979800735,-3.78025488954978,
-9.90494107374827));
#26193=CARTESIAN_POINT('Ctrl Pts',(-41.2927947172303,-3.78068932547453,
-9.90670364958125));
#26194=CARTESIAN_POINT('',(-41.3,-3.43999690767065,-8.52446017500325));
#26195=CARTESIAN_POINT('',(-41.3,-2.10739801921515,-3.11789395415524));
#26196=CARTESIAN_POINT('',(-40.8,-3.55965473981442,-9.00993108371627));
#26197=CARTESIAN_POINT('',(-41.05,-3.49982582374253,-8.76719562935976));
#26198=CARTESIAN_POINT('',(-41.3,-3.55965473981442,-9.00993108371627));
#26199=CARTESIAN_POINT('Origin',(-24.9,-5.96274352296443,-9.06428794965443));
#26200=CARTESIAN_POINT('',(-16.2963973586152,-6.0053809436503,-8.73909541646189));
#26201=CARTESIAN_POINT('',(-41.2927947172303,-6.0053809436503,-8.73909541646189));
#26202=CARTESIAN_POINT('',(-24.9,-6.0053809436503,-8.73909541646189));
#26203=CARTESIAN_POINT('Ctrl Pts',(-41.2927947172303,-6.0053809436503,-8.73909541646189));
#26204=CARTESIAN_POINT('Ctrl Pts',(-40.8162222946065,-5.96371871143227,
-9.05685025752629));
#26205=CARTESIAN_POINT('Ctrl Pts',(-40.3,-5.92010610227855,-9.38948048284697));
#26206=CARTESIAN_POINT('Ctrl Pts',(-15.8,-5.92010610227855,-9.38948048284698));
#26207=CARTESIAN_POINT('Ctrl Pts',(-15.967063448461,-5.94833453393571,-9.17418427001376));
#26208=CARTESIAN_POINT('Ctrl Pts',(-16.1329130514352,-5.97679716143211,
-8.95710186240145));
#26209=CARTESIAN_POINT('Ctrl Pts',(-16.2963973586152,-6.0053809436503,-8.73909541646189));
#26210=CARTESIAN_POINT('Origin',(-24.9,-8.27946977552996,-7.01184758754715));
#26211=CARTESIAN_POINT('',(-41.2927947172303,-7.95150888889516,-7.01497650503582));
#26212=CARTESIAN_POINT('Ctrl Pts',(-40.3,-8.60743066216474,-7.00871867005847));
#26213=CARTESIAN_POINT('Ctrl Pts',(-40.816222294603,-8.27196876657345,-7.01191915107519));
#26214=CARTESIAN_POINT('Ctrl Pts',(-41.2927947172303,-7.95150888889516,
-7.01497650503582));
#26215=CARTESIAN_POINT('',(-16.2963973586152,-7.95150888889517,-7.01497650503582));
#26216=CARTESIAN_POINT('',(-24.9,-7.95150888889517,-7.01497650503582));
#26217=CARTESIAN_POINT('Ctrl Pts',(-16.2963973586152,-7.95150888889517,
-7.01497650503582));
#26218=CARTESIAN_POINT('Ctrl Pts',(-16.1329130514351,-8.17137121660771,
-7.01287890404035));
#26219=CARTESIAN_POINT('Ctrl Pts',(-15.9670634484609,-8.39030163968482,
-7.01079019389995));
#26220=CARTESIAN_POINT('Ctrl Pts',(-15.8,-8.60743066216474,-7.00871867005847));
#26221=CARTESIAN_POINT('Origin',(-16.05,0.,0.));
#26222=CARTESIAN_POINT('',(-16.3,-7.94910173040956,-7.01225938479173));
#26223=CARTESIAN_POINT('Ctrl Pts',(-16.2963973586152,-7.95150888889512,
-7.01497650503579));
#26224=CARTESIAN_POINT('Ctrl Pts',(-16.2981989900367,-7.95030510515574,
-7.01361771408482));
#26225=CARTESIAN_POINT('Ctrl Pts',(-16.3,-7.94910173040954,-7.01225938479171));
#26226=CARTESIAN_POINT('',(-16.3,-6.0029737851647,-8.7363782962178));
#26227=CARTESIAN_POINT('Origin',(-16.3,0.,0.));
#26228=CARTESIAN_POINT('Ctrl Pts',(-16.3,-6.00297378516469,-8.73637829621777));
#26229=CARTESIAN_POINT('Ctrl Pts',(-16.2981989900367,-6.0041771599109,-8.73773662551088));
#26230=CARTESIAN_POINT('Ctrl Pts',(-16.2963973586151,-6.00538094365029,
-8.73909541646186));
#26231=CARTESIAN_POINT('Origin',(-41.3,-6.52022206549856,-9.32023091004648));
#26232=CARTESIAN_POINT('',(-16.3,-5.39291354648921,-8.0477626381556));
#26233=CARTESIAN_POINT('',(-16.3,-6.52022206549856,-9.32023091004648));
#26234=CARTESIAN_POINT('',(-40.8,-5.39291354648921,-8.0477626381556));
#26235=CARTESIAN_POINT('',(-41.3,-5.39291354648921,-8.0477626381556));
#26236=CARTESIAN_POINT('',(-41.3,-5.06135221736881,-7.67350726407005));
#26237=CARTESIAN_POINT('',(-40.625,-5.50896001168135,-8.17875201908555));
#26238=CARTESIAN_POINT('',(-41.3,-6.0029737851647,-8.73637829621779));
#26239=CARTESIAN_POINT('',(-41.3,-0.443001249114668,-2.46046666651991));
#26240=CARTESIAN_POINT('Ctrl Pts',(-41.2927947172303,-6.0053809436503,-8.73909541646189));
#26241=CARTESIAN_POINT('Ctrl Pts',(-41.2963979800734,-6.00417715991092,
-8.73773662551092));
#26242=CARTESIAN_POINT('Ctrl Pts',(-41.3,-6.0029737851647,-8.73637829621779));
#26243=CARTESIAN_POINT('Origin',(-16.3,-6.92963177861631,-7.821937318388));
#26244=CARTESIAN_POINT('',(-16.3,-7.33904149173407,-6.32364372672953));
#26245=CARTESIAN_POINT('',(-16.3,-7.33904149173407,-6.32364372672953));
#26246=CARTESIAN_POINT('',(-16.3,-5.39291354648921,-8.0477626381556));
#26247=CARTESIAN_POINT('Origin',(-41.3,-7.33904149173407,-6.32364372672953));
#26248=CARTESIAN_POINT('',(-41.3,-7.94910173040956,-7.01225938479172));
#26249=CARTESIAN_POINT('Ctrl Pts',(-41.3,-7.94910173040956,-7.01225938479172));
#26250=CARTESIAN_POINT('Ctrl Pts',(-41.2963979800735,-7.95030510515576,
-7.01361771408483));
#26251=CARTESIAN_POINT('Ctrl Pts',(-41.2927947172303,-7.95150888889516,
-7.01497650503582));
#26252=CARTESIAN_POINT('',(-41.3,-7.00748016261367,-5.94938835264399));
#26253=CARTESIAN_POINT('',(-41.3,-1.82547493485485,-0.100113619148405));
#26254=CARTESIAN_POINT('',(-40.8,-7.33904149173407,-6.32364372672953));
#26255=CARTESIAN_POINT('',(-41.05,-7.17326082717387,-6.13651603968676));
#26256=CARTESIAN_POINT('',(-41.3,-7.33904149173407,-6.32364372672953));
#26257=CARTESIAN_POINT('Origin',(-41.05,4.65,9.35));
#26258=CARTESIAN_POINT('',(-41.3,-1.3,9.1));
#26259=CARTESIAN_POINT('',(-40.8,-1.3,9.6));
#26260=CARTESIAN_POINT('',(-40.625,-1.3,9.775));
#26261=CARTESIAN_POINT('',(-40.8,1.3,9.6));
#26262=CARTESIAN_POINT('',(-40.8,4.65,9.6));
#26263=CARTESIAN_POINT('',(-41.3,1.3,9.1));
#26264=CARTESIAN_POINT('',(-41.05,1.3,9.35));
#26265=CARTESIAN_POINT('',(-41.3,4.65,9.1));
#26266=CARTESIAN_POINT('Origin',(-41.3,-1.3,9.6));
#26267=CARTESIAN_POINT('',(-16.3,-1.3,9.6));
#26268=CARTESIAN_POINT('',(-41.3,-1.3,9.6));
#26269=CARTESIAN_POINT('',(-16.3,1.3,9.6));
#26270=CARTESIAN_POINT('',(-16.3,-1.3,9.6));
#26271=CARTESIAN_POINT('',(-41.3,1.3,9.6));
#26272=CARTESIAN_POINT('Origin',(-41.05,-0.765336496446259,10.1578510226473));
#26273=CARTESIAN_POINT('',(-41.3,-5.38007369894747,7.45350970978731));
#26274=CARTESIAN_POINT('',(-40.8,-5.61243528496935,7.89623772261392));
#26275=CARTESIAN_POINT('',(-40.625,-5.69376184007701,8.05119252710323));
#26276=CARTESIAN_POINT('',(-40.8,-3.310249618271,9.10451796992771));
#26277=CARTESIAN_POINT('',(-40.8,-0.8815172894572,10.3792150290606));
#26278=CARTESIAN_POINT('',(-41.3,-3.07788803224912,8.66178995710111));
#26279=CARTESIAN_POINT('',(-41.05,-3.19406882526006,8.88315396351441));
#26280=CARTESIAN_POINT('',(-41.3,-0.649155703435317,9.93648701623395));
#26281=CARTESIAN_POINT('Origin',(-41.3,-5.61243528496935,7.89623772261392));
#26282=CARTESIAN_POINT('',(-16.3,-5.61243528496935,7.89623772261392));
#26283=CARTESIAN_POINT('',(-41.3,-5.61243528496935,7.89623772261392));
#26284=CARTESIAN_POINT('',(-16.3,-3.310249618271,9.10451796992771));
#26285=CARTESIAN_POINT('',(-16.3,-5.61243528496935,7.89623772261392));
#26286=CARTESIAN_POINT('',(-41.3,-3.310249618271,9.10451796992771));
#26287=CARTESIAN_POINT('Origin',(-41.05,-6.35384418214366,7.25425891222178));
#26288=CARTESIAN_POINT('',(-41.3,-8.22763735038278,4.09951016959177));
#26289=CARTESIAN_POINT('',(-40.8,-8.6391292833296,4.38354254295734));
#26290=CARTESIAN_POINT('',(-40.625,-8.783151459861,4.4829538736353));
#26291=CARTESIAN_POINT('',(-40.8,-7.1621609418286,6.52330059428085));
#26292=CARTESIAN_POINT('',(-40.8,-6.55959014861707,7.39627509890457));
#26293=CARTESIAN_POINT('',(-41.3,-6.75066900888177,6.23926822091527));
#26294=CARTESIAN_POINT('',(-41.05,-6.95641497535519,6.38128440759806));
#26295=CARTESIAN_POINT('',(-41.3,-6.14809821567024,7.11224272553899));
#26296=CARTESIAN_POINT('Origin',(-41.3,-8.6391292833296,4.38354254295734));
#26297=CARTESIAN_POINT('',(-16.3,-8.6391292833296,4.38354254295734));
#26298=CARTESIAN_POINT('',(-41.3,-8.6391292833296,4.38354254295734));
#26299=CARTESIAN_POINT('',(-16.3,-7.1621609418286,6.52330059428085));
#26300=CARTESIAN_POINT('',(-16.3,-8.6391292833296,4.38354254295734));
#26301=CARTESIAN_POINT('',(-41.3,-7.1621609418286,6.52330059428085));
#26302=CARTESIAN_POINT('Origin',(-41.05,-9.2831726311618,1.11594370258557));
#26303=CARTESIAN_POINT('',(-41.3,-9.19034843862421,-0.193637746004029));
#26304=CARTESIAN_POINT('',(-40.8,-9.68670287567324,-0.133369405876367));
#26305=CARTESIAN_POINT('',(-40.625,-9.8604269286404,-0.112275486831686));
#26306=CARTESIAN_POINT('',(-40.8,-9.3733075070094,2.44767366677857));
#26307=CARTESIAN_POINT('',(-40.8,-9.53134984968631,1.1460778726494));
#26308=CARTESIAN_POINT('',(-41.3,-8.87695306996037,2.38740532665091));
#26309=CARTESIAN_POINT('',(-41.05,-9.12513028848489,2.41753949671474));
#26310=CARTESIAN_POINT('',(-41.3,-9.03499541263729,1.08580953252174));
#26311=CARTESIAN_POINT('Origin',(-41.3,-9.68670287567324,-0.133369405876367));
#26312=CARTESIAN_POINT('',(-16.3,-9.68670287567324,-0.133369405876367));
#26313=CARTESIAN_POINT('',(-41.3,-9.68670287567324,-0.133369405876367));
#26314=CARTESIAN_POINT('',(-16.3,-9.3733075070094,2.44767366677857));
#26315=CARTESIAN_POINT('',(-16.3,-9.68670287567324,-0.133369405876367));
#26316=CARTESIAN_POINT('',(-41.3,-9.3733075070094,2.44767366677857));
#26317=CARTESIAN_POINT('Origin',(-41.05,-7.8454621751844,-5.68059129593133));
#26318=CARTESIAN_POINT('',(-41.3,-8.04766145528198,-4.44242558757811));
#26319=CARTESIAN_POINT('',(-40.8,-8.51516957662469,-4.61972803109938));
#26320=CARTESIAN_POINT('',(-40.625,-8.67879741909464,-4.68178388633183));
#26321=CARTESIAN_POINT('',(-40.8,-9.43714228293528,-2.1886858001173));
#26322=CARTESIAN_POINT('',(-40.8,-8.07921623585575,-5.76924251769197));
#26323=CARTESIAN_POINT('',(-41.3,-8.96963416159257,-2.01138335659603));
#26324=CARTESIAN_POINT('',(-41.05,-9.20338822226393,-2.10003457835667));
#26325=CARTESIAN_POINT('',(-41.3,-7.61170811451305,-5.5919400741707));
#26326=CARTESIAN_POINT('Origin',(-41.3,-8.51516957662469,-4.61972803109938));
#26327=CARTESIAN_POINT('',(-16.3,-8.51516957662469,-4.61972803109938));
#26328=CARTESIAN_POINT('',(-41.3,-8.51516957662469,-4.61972803109938));
#26329=CARTESIAN_POINT('',(-16.3,-9.43714228293528,-2.1886858001173));
#26330=CARTESIAN_POINT('',(-16.3,-8.51516957662469,-4.61972803109938));
#26331=CARTESIAN_POINT('',(-41.3,-9.43714228293528,-2.1886858001173));
#26332=CARTESIAN_POINT('Origin',(-41.05,-2.74424266556362,-10.0602837396162));
#26333=CARTESIAN_POINT('',(-40.8,-2.91002333012382,-10.2474114266589));
#26334=CARTESIAN_POINT('',(-41.3,-2.57846200100342,-9.87315605257338));
#26335=CARTESIAN_POINT('Origin',(-41.3,-5.39291354648921,-8.0477626381556));
#26336=CARTESIAN_POINT('Origin',(-41.05,3.38996918821927,-10.4653775806365));
#26337=CARTESIAN_POINT('',(-40.8,3.33014027214738,-10.708113034993));
#26338=CARTESIAN_POINT('',(-41.3,3.44979810429116,-10.22264212628));
#26339=CARTESIAN_POINT('Origin',(-41.3,-1.03520601450669,-9.63215181086392));
#26340=CARTESIAN_POINT('Origin',(-41.05,7.8651721103966,-7.69123440523069));
#26341=CARTESIAN_POINT('',(-40.8,7.92500102646849,-7.9339698595872));
#26342=CARTESIAN_POINT('',(-41.3,7.80534319432471,-7.44849895087418));
#26343=CARTESIAN_POINT('Origin',(-41.3,3.55965473981442,-9.00993108371628));
#26344=CARTESIAN_POINT('',(-16.3,3.55965473981442,-9.00993108371628));
#26345=CARTESIAN_POINT('Origin',(-41.05,9.65615104353926,-3.93686725118344));
#26346=CARTESIAN_POINT('',(-40.8,9.82193170809946,-4.12399493822621));
#26347=CARTESIAN_POINT('',(-41.3,9.49037037897906,-3.74973956414066));
#26348=CARTESIAN_POINT('Origin',(-41.3,7.33904149173406,-6.32364372672954));
#26349=CARTESIAN_POINT('Origin',(-41.05,9.63934156303286,-0.950520091764082));
#26350=CARTESIAN_POINT('',(-40.8,9.87309562370421,-1.03917131352472));
#26351=CARTESIAN_POINT('',(-41.3,9.40558750236151,-0.861868870003448));
#26352=CARTESIAN_POINT('Origin',(-41.3,9.43714228293528,-2.18868580011731));
#26353=CARTESIAN_POINT('Origin',(-41.05,9.28048331447181,1.13809221818897));
#26354=CARTESIAN_POINT('',(-40.8,9.52866053299632,1.16822638825281));
#26355=CARTESIAN_POINT('',(-41.3,9.03230609594729,1.10795804812514));
#26356=CARTESIAN_POINT('Origin',(-41.3,9.3733075070094,2.44767366677856));
#26357=CARTESIAN_POINT('Origin',(-41.05,9.03595411006772,3.36855185165083));
#26358=CARTESIAN_POINT('',(-40.8,9.24170007654113,3.51056803833362));
#26359=CARTESIAN_POINT('',(-41.3,8.8302081435943,3.22653566496804));
#26360=CARTESIAN_POINT('Origin',(-41.3,7.1621609418286,6.52330059428085));
#26361=CARTESIAN_POINT('Origin',(-24.9,-9.49213183011501,-5.25500329920184));
#26362=CARTESIAN_POINT('',(-16.2963973586152,-9.37876088562945,-4.94724501380016));
#26363=CARTESIAN_POINT('',(-41.2927947172303,-9.37876088562945,-4.94724501380016));
#26364=CARTESIAN_POINT('',(-24.9,-9.37876088562945,-4.94724501380016));
#26365=CARTESIAN_POINT('Ctrl Pts',(-41.2927947172303,-9.37876088562945,
-4.94724501380016));
#26366=CARTESIAN_POINT('Ctrl Pts',(-40.8162222946069,-9.48953884874146,
-5.24796435721168));
#26367=CARTESIAN_POINT('Ctrl Pts',(-40.3,-9.60550277460057,-5.5627615846035));
#26368=CARTESIAN_POINT('Ctrl Pts',(-15.8,-9.60550277460058,-5.56276158460351));
#26369=CARTESIAN_POINT('Ctrl Pts',(-15.9670634484609,-9.53044467054936,
-5.35900784934866));
#26370=CARTESIAN_POINT('Ctrl Pts',(-16.1329130514351,-9.45476385051144,
-5.15356368093011));
#26371=CARTESIAN_POINT('Ctrl Pts',(-16.2963973586152,-9.37876088562945,
-4.94724501380016));
#26372=CARTESIAN_POINT('Origin',(-24.9,-10.589674454729,-2.36102124043076));
#26373=CARTESIAN_POINT('',(-41.2927947172303,-10.30073359194,-2.51620278281808));
#26374=CARTESIAN_POINT('Ctrl Pts',(-40.3,-10.8786153175179,-2.20583969804344));
#26375=CARTESIAN_POINT('Ctrl Pts',(-40.8162222946029,-10.5830658983798,
-2.36457049946365));
#26376=CARTESIAN_POINT('Ctrl Pts',(-41.2927947172303,-10.30073359194,-2.51620278281808));
#26377=CARTESIAN_POINT('',(-16.2963973586152,-10.30073359194,-2.51620278281808));
#26378=CARTESIAN_POINT('',(-24.9,-10.30073359194,-2.51620278281808));
#26379=CARTESIAN_POINT('Ctrl Pts',(-16.2963973586152,-10.30073359194,-2.51620278281808));
#26380=CARTESIAN_POINT('Ctrl Pts',(-16.1329130514352,-10.4944372110389,
-2.41217033102977));
#26381=CARTESIAN_POINT('Ctrl Pts',(-15.9670634484611,-10.6873198013493,
-2.30857882938089));
#26382=CARTESIAN_POINT('Ctrl Pts',(-15.8,-10.8786153175179,-2.20583969804343));
#26383=CARTESIAN_POINT('Origin',(-16.05,0.,0.));
#26384=CARTESIAN_POINT('',(-16.3,-10.2973394502156,-2.51491555465257));
#26385=CARTESIAN_POINT('Ctrl Pts',(-16.2963973586152,-10.3007335919401,
-2.51620278281809));
#26386=CARTESIAN_POINT('Ctrl Pts',(-16.2981989900368,-10.2990362327336,
-2.51555905938076));
#26387=CARTESIAN_POINT('Ctrl Pts',(-16.3000000000001,-10.2973394502156,
-2.51491555465257));
#26388=CARTESIAN_POINT('',(-16.3,-9.37536674390501,-4.94595778563465));
#26389=CARTESIAN_POINT('Origin',(-16.3,0.,0.));
#26390=CARTESIAN_POINT('Ctrl Pts',(-16.3000000000001,-9.37536674390505,
-4.94595778563467));
#26391=CARTESIAN_POINT('Ctrl Pts',(-16.2981989900368,-9.37706352642298,
-4.94660129036286));
#26392=CARTESIAN_POINT('Ctrl Pts',(-16.2963973586152,-9.37876088562949,
-4.94724501380019));
#26393=CARTESIAN_POINT('Origin',(-41.3,-10.1046971891899,-5.22255633907169));
#26394=CARTESIAN_POINT('',(-16.3,-10.1046971891899,-5.22255633907169));
#26395=CARTESIAN_POINT('',(-41.3,-9.375366743905,-4.94595778563464));
#26396=CARTESIAN_POINT('',(-41.3,-0.18830193536388,-1.46176368294326));
#26397=CARTESIAN_POINT('Ctrl Pts',(-41.2927947172303,-9.37876088562945,
-4.94724501380016));
#26398=CARTESIAN_POINT('Ctrl Pts',(-41.2963979800734,-9.37706352642294,
-4.94660129036284));
#26399=CARTESIAN_POINT('Ctrl Pts',(-41.3,-9.375366743905,-4.94595778563464));
#26400=CARTESIAN_POINT('Origin',(-16.3,-9.77091973606259,-3.7056210695945));
#26401=CARTESIAN_POINT('',(-16.3,-9.43714228293528,-2.1886858001173));
#26402=CARTESIAN_POINT('Origin',(-41.3,-9.43714228293528,-2.1886858001173));
#26403=CARTESIAN_POINT('',(-41.3,-10.2973394502156,-2.51491555465256));
#26404=CARTESIAN_POINT('Ctrl Pts',(-41.3,-10.2973394502156,-2.51491555465256));
#26405=CARTESIAN_POINT('Ctrl Pts',(-41.2963979800735,-10.2990362327335,
-2.51555905938075));
#26406=CARTESIAN_POINT('Ctrl Pts',(-41.2927947172303,-10.30073359194,-2.51620278281808));
#26407=CARTESIAN_POINT('',(-41.3,-0.315510835391869,1.27069270202498));
#26408=CARTESIAN_POINT('Origin',(-24.9,-10.8469871275755,-0.241860722557092));
#26409=CARTESIAN_POINT('',(-16.2963973586152,-10.6035797350322,-0.0220403992424092));
#26410=CARTESIAN_POINT('',(-41.2927947172303,-10.6035797350322,-0.0220403992424095));
#26411=CARTESIAN_POINT('',(-24.9,-10.6035797350322,-0.0220403992424092));
#26412=CARTESIAN_POINT('Ctrl Pts',(-41.2927947172303,-10.6035797350322,
-0.0220403992424095));
#26413=CARTESIAN_POINT('Ctrl Pts',(-40.8162222946062,-10.8414199971447,
-0.236833067486949));
#26414=CARTESIAN_POINT('Ctrl Pts',(-40.3,-11.0903945201189,-0.461681045871771));
#26415=CARTESIAN_POINT('Ctrl Pts',(-15.8,-11.0903945201189,-0.461681045871777));
#26416=CARTESIAN_POINT('Ctrl Pts',(-15.967063448461,-10.9292447874491,-0.316147313443195));
#26417=CARTESIAN_POINT('Ctrl Pts',(-16.1329130514351,-10.7667580836948,
-0.169406167332626));
#26418=CARTESIAN_POINT('Ctrl Pts',(-16.2963973586152,-10.6035797350322,
-0.0220403992424079));
#26419=CARTESIAN_POINT('Origin',(-24.9,-10.4739123357613,2.83068661947789));
#26420=CARTESIAN_POINT('',(-41.2927947172303,-10.2901843663683,2.55900267341253));
#26421=CARTESIAN_POINT('Ctrl Pts',(-40.3,-10.6576403051544,3.10237056554323));
#26422=CARTESIAN_POINT('Ctrl Pts',(-40.8162222946031,-10.4697101726372,
2.82447275741129));
#26423=CARTESIAN_POINT('Ctrl Pts',(-41.2927947172303,-10.2901843663683,
2.55900267341253));
#26424=CARTESIAN_POINT('',(-16.2963973586152,-10.2901843663683,2.55900267341253));
#26425=CARTESIAN_POINT('',(-24.9,-10.2901843663683,2.55900267341253));
#26426=CARTESIAN_POINT('Ctrl Pts',(-16.2963973586152,-10.2901843663683,
2.55900267341253));
#26427=CARTESIAN_POINT('Ctrl Pts',(-16.1329130514351,-10.4133541120997,
2.741137395016));
#26428=CARTESIAN_POINT('Ctrl Pts',(-15.967063448461,-10.5360017926907,2.92250012355862));
#26429=CARTESIAN_POINT('Ctrl Pts',(-15.8,-10.6576403051544,3.10237056554324));
#26430=CARTESIAN_POINT('Origin',(-16.05,0.,0.));
#26431=CARTESIAN_POINT('',(-16.3,-10.2865807983703,2.55856512103953));
#26432=CARTESIAN_POINT('Ctrl Pts',(-16.2963973586152,-10.2901843663683,
2.55900267341253));
#26433=CARTESIAN_POINT('Ctrl Pts',(-16.2981989900368,-10.2883822762335,
2.55878386005441));
#26434=CARTESIAN_POINT('Ctrl Pts',(-16.3000000000001,-10.2865807983703,
2.55856512103953));
#26435=CARTESIAN_POINT('',(-16.3,-10.5999761670341,-0.0224779516154086));
#26436=CARTESIAN_POINT('Origin',(-16.3,0.,0.));
#26437=CARTESIAN_POINT('Ctrl Pts',(-16.3000000000001,-10.5999761670342,
-0.022477951615407));
#26438=CARTESIAN_POINT('Ctrl Pts',(-16.2981989900368,-10.6017776448974,
-0.022259212600522));
#26439=CARTESIAN_POINT('Ctrl Pts',(-16.2963973586152,-10.6035797350322,
-0.022040399242408));
#26440=CARTESIAN_POINT('Origin',(-41.3,-11.3743079616399,0.0715429505576823));
#26441=CARTESIAN_POINT('',(-16.3,-11.3743079616399,0.0715429505576823));
#26442=CARTESIAN_POINT('',(-41.3,-10.5999761670341,-0.0224779516154098));
#26443=CARTESIAN_POINT('',(-41.3,-0.542507006806888,-1.24367580324692));
#26444=CARTESIAN_POINT('Ctrl Pts',(-41.2927947172303,-10.6035797350322,
-0.0220403992424095));
#26445=CARTESIAN_POINT('Ctrl Pts',(-41.2963979800735,-10.6017776448973,
-0.0222592126005259));
#26446=CARTESIAN_POINT('Ctrl Pts',(-41.3,-10.5999761670341,-0.0224779516154095));
#26447=CARTESIAN_POINT('Origin',(-16.3,-10.3738077343247,1.25960830866813));
#26448=CARTESIAN_POINT('',(-16.3,-9.3733075070094,2.44767366677857));
#26449=CARTESIAN_POINT('Origin',(-41.3,-9.3733075070094,2.44767366677857));
#26450=CARTESIAN_POINT('',(-41.3,-10.2865807983703,2.55856512103953));
#26451=CARTESIAN_POINT('Ctrl Pts',(-41.3,-10.2865807983703,2.55856512103953));
#26452=CARTESIAN_POINT('Ctrl Pts',(-41.2963979800734,-10.2883822762335,
2.55878386005442));
#26453=CARTESIAN_POINT('Ctrl Pts',(-41.2927947172303,-10.2901843663683,
2.55900267341253));
#26454=CARTESIAN_POINT('',(-41.3,0.614690904840299,1.23491109119099));
#26455=CARTESIAN_POINT('Origin',(-24.9,-9.71692839447407,4.8266892308878));
#26456=CARTESIAN_POINT('',(-16.2963973586152,-9.39924625412754,4.90821340516617));
#26457=CARTESIAN_POINT('',(-41.2927947172303,-9.39924625412754,4.90821340516618));
#26458=CARTESIAN_POINT('',(-24.9,-9.39924625412754,4.90821340516617));
#26459=CARTESIAN_POINT('Ctrl Pts',(-41.2927947172303,-9.39924625412754,
4.90821340516618));
#26460=CARTESIAN_POINT('Ctrl Pts',(-40.8162222946068,-9.70966247747601,
4.82855382385169));
#26461=CARTESIAN_POINT('Ctrl Pts',(-40.3,-10.0346105348206,4.74516505660943));
#26462=CARTESIAN_POINT('Ctrl Pts',(-15.8,-10.0346105348206,4.74516505660943));
#26463=CARTESIAN_POINT('Ctrl Pts',(-15.967063448461,-9.8242866352221,4.79913876198384));
#26464=CARTESIAN_POINT('Ctrl Pts',(-16.1329130514352,-9.61221779340458,
4.85356025763508));
#26465=CARTESIAN_POINT('Ctrl Pts',(-16.2963973586152,-9.39924625412754,
4.90821340516617));
#26466=CARTESIAN_POINT('Origin',(-24.9,-7.95870312499775,7.37391828833598));
#26467=CARTESIAN_POINT('',(-41.2927947172303,-7.92227791262653,7.04797145648968));
#26468=CARTESIAN_POINT('Ctrl Pts',(-40.3,-7.99512833736897,7.69986512018227));
#26469=CARTESIAN_POINT('Ctrl Pts',(-40.8162222946026,-7.95787002002895,
7.36646334415037));
#26470=CARTESIAN_POINT('Ctrl Pts',(-41.2927947172303,-7.92227791262653,
7.04797145648968));
#26471=CARTESIAN_POINT('',(-16.2963973586152,-7.92227791262653,7.04797145648968));
#26472=CARTESIAN_POINT('',(-24.9,-7.92227791262653,7.04797145648968));
#26473=CARTESIAN_POINT('Ctrl Pts',(-16.2963973586152,-7.92227791262653,
7.04797145648968));
#26474=CARTESIAN_POINT('Ctrl Pts',(-16.1329130514351,-7.94669708059969,
7.26648357815028));
#26475=CARTESIAN_POINT('Ctrl Pts',(-15.9670634484609,-7.9710127459125,7.48406951813532));
#26476=CARTESIAN_POINT('Ctrl Pts',(-15.8,-7.99512833736897,7.69986512018228));
#26477=CARTESIAN_POINT('Origin',(-16.05,0.,0.));
#26478=CARTESIAN_POINT('',(-16.3,-7.91929045235552,7.04590936155374));
#26479=CARTESIAN_POINT('Ctrl Pts',(-16.2963973586152,-7.92227791262651,
7.04797145648969));
#26480=CARTESIAN_POINT('Ctrl Pts',(-16.2981989900368,-7.92078392869575,
7.0469402338395));
#26481=CARTESIAN_POINT('Ctrl Pts',(-16.3,-7.91929045235552,7.04590936155376));
#26482=CARTESIAN_POINT('',(-16.3,-9.39625879385653,4.90615131023023));
#26483=CARTESIAN_POINT('Origin',(-16.3,0.,0.));
#26484=CARTESIAN_POINT('Ctrl Pts',(-16.3000000000001,-9.39625879385658,
4.90615131023027));
#26485=CARTESIAN_POINT('Ctrl Pts',(-16.2981989900368,-9.39775227019682,
4.90718218251601));
#26486=CARTESIAN_POINT('Ctrl Pts',(-16.2963973586152,-9.39924625412759,
4.9082134051662));
#26487=CARTESIAN_POINT('Origin',(-41.3,-10.0382018553488,5.34925261240031));
#26488=CARTESIAN_POINT('',(-16.3,-10.0382018553488,5.34925261240031));
#26489=CARTESIAN_POINT('',(-41.3,-9.39625879385652,4.90615131023023));
#26490=CARTESIAN_POINT('',(-41.3,-1.79864006238694,-0.338106249747072));
#26491=CARTESIAN_POINT('Ctrl Pts',(-41.2927947172303,-9.39924625412754,
4.90821340516618));
#26492=CARTESIAN_POINT('Ctrl Pts',(-41.2963979800734,-9.39775227019676,
4.90718218251598));
#26493=CARTESIAN_POINT('Ctrl Pts',(-41.3,-9.39625879385652,4.90615131023023));
#26494=CARTESIAN_POINT('Origin',(-16.3,-8.60018139858871,5.93627660334058));
#26495=CARTESIAN_POINT('',(-16.3,-7.1621609418286,6.52330059428085));
#26496=CARTESIAN_POINT('Origin',(-41.3,-7.1621609418286,6.52330059428085));
#26497=CARTESIAN_POINT('',(-41.3,-7.91929045235552,7.04590936155374));
#26498=CARTESIAN_POINT('Ctrl Pts',(-41.3,-7.91929045235552,7.04590936155374));
#26499=CARTESIAN_POINT('Ctrl Pts',(-41.2963979800734,-7.92078392869579,
7.0469402338395));
#26500=CARTESIAN_POINT('Ctrl Pts',(-41.2927947172303,-7.92227791262653,
7.04797145648968));
#26501=CARTESIAN_POINT('',(-41.3,0.377864565123671,1.31879676685495));
#26502=CARTESIAN_POINT('Origin',(-24.9,-6.36083846788016,8.78950284944722));
#26503=CARTESIAN_POINT('',(-16.2963973586152,-6.04165872959902,8.71405466883491));
#26504=CARTESIAN_POINT('',(-41.2927947172303,-6.04165872959902,8.71405466883491));
#26505=CARTESIAN_POINT('',(-24.9,-6.04165872959902,8.71405466883491));
#26506=CARTESIAN_POINT('Ctrl Pts',(-41.2927947172303,-6.04165872959902,
8.71405466883491));
#26507=CARTESIAN_POINT('Ctrl Pts',(-40.8162222946063,-6.35353829833592,
8.78777722452741));
#26508=CARTESIAN_POINT('Ctrl Pts',(-40.3,-6.6800182061613,8.86495103005952));
#26509=CARTESIAN_POINT('Ctrl Pts',(-15.8,-6.68001820616131,8.86495103005953));
#26510=CARTESIAN_POINT('Ctrl Pts',(-15.967063448461,-6.46870281035439,8.8149999829321));
#26511=CARTESIAN_POINT('Ctrl Pts',(-16.1329130514352,-6.25563424642735,
8.76463451932045));
#26512=CARTESIAN_POINT('Ctrl Pts',(-16.2963973586152,-6.04165872959902,
8.71405466883491));
#26513=CARTESIAN_POINT('Origin',(-24.9,-3.62025094106724,10.2278741426851));
#26514=CARTESIAN_POINT('',(-41.2927947172303,-3.73947306290067,9.9223349161487));
#26515=CARTESIAN_POINT('Ctrl Pts',(-40.3,-3.50102881923381,10.5334133692215));
#26516=CARTESIAN_POINT('Ctrl Pts',(-40.8162222946038,-3.62297774856226,
10.2208859542505));
#26517=CARTESIAN_POINT('Ctrl Pts',(-41.2927947172303,-3.73947306290067,
9.9223349161487));
#26518=CARTESIAN_POINT('',(-16.2963973586152,-3.73947306290067,9.9223349161487));
#26519=CARTESIAN_POINT('',(-24.9,-3.73947306290067,9.9223349161487));
#26520=CARTESIAN_POINT('Ctrl Pts',(-16.2963973586152,-3.73947306290067,
9.9223349161487));
#26521=CARTESIAN_POINT('Ctrl Pts',(-16.1329130514351,-3.65954751601581,
10.1271659441505));
#26522=CARTESIAN_POINT('Ctrl Pts',(-15.9670634484609,-3.57996074016283,
10.3311287789222));
#26523=CARTESIAN_POINT('Ctrl Pts',(-15.8,-3.50102881923381,10.5334133692215));
#26524=CARTESIAN_POINT('Origin',(-16.05,0.,0.));
#26525=CARTESIAN_POINT('',(-16.3,-3.737786101502,9.91912067974871));
#26526=CARTESIAN_POINT('Ctrl Pts',(-16.2963973586153,-3.7394730629007,9.92233491614877));
#26527=CARTESIAN_POINT('Ctrl Pts',(-16.2981989900368,-3.73862943888804,
9.92072752488807));
#26528=CARTESIAN_POINT('Ctrl Pts',(-16.3000000000001,-3.73778610150201,
9.91912067974877));
#26529=CARTESIAN_POINT('',(-16.3,-6.03997176820034,8.71084043243491));
#26530=CARTESIAN_POINT('Origin',(-16.3,0.,0.));
#26531=CARTESIAN_POINT('Ctrl Pts',(-16.3000000000001,-6.03997176820037,
8.71084043243496));
#26532=CARTESIAN_POINT('Ctrl Pts',(-16.2981989900368,-6.0408151055864,8.71244727757426));
#26533=CARTESIAN_POINT('Ctrl Pts',(-16.2963973586152,-6.04165872959905,
8.71405466883496));
#26534=CARTESIAN_POINT('Origin',(-41.3,-6.40246467744376,9.40151296622437));
#26535=CARTESIAN_POINT('',(-16.3,-6.40246467744376,9.40151296622437));
#26536=CARTESIAN_POINT('',(-41.3,-6.03997176820034,8.71084043243491));
#26537=CARTESIAN_POINT('',(-41.3,-2.63215033423403,2.21777917666555));
#26538=CARTESIAN_POINT('Ctrl Pts',(-41.2927947172303,-6.04165872959902,
8.71405466883491));
#26539=CARTESIAN_POINT('Ctrl Pts',(-41.2963979800735,-6.04081510558637,
8.71244727757421));
#26540=CARTESIAN_POINT('Ctrl Pts',(-41.3,-6.03997176820034,8.71084043243491));
#26541=CARTESIAN_POINT('Origin',(-16.3,-4.85635714785738,9.25301546807604));
#26542=CARTESIAN_POINT('',(-16.3,-3.310249618271,9.10451796992771));
#26543=CARTESIAN_POINT('Origin',(-41.3,-3.310249618271,9.10451796992771));
#26544=CARTESIAN_POINT('',(-41.3,-3.73778610150199,9.9191206797487));
#26545=CARTESIAN_POINT('Ctrl Pts',(-41.3,-3.73778610150199,9.9191206797487));
#26546=CARTESIAN_POINT('Ctrl Pts',(-41.2963979800734,-3.73862943888803,
9.92072752488801));
#26547=CARTESIAN_POINT('Ctrl Pts',(-41.2927947172303,-3.73947306290067,
9.9223349161487));
#26548=CARTESIAN_POINT('',(-41.3,0.0650500287015215,2.67342180217412));
#26549=CARTESIAN_POINT('Origin',(-24.9,-1.54755710470837,10.7387472901904));
#26550=CARTESIAN_POINT('',(-16.2963973586152,-1.3,10.5236110236165));
#26551=CARTESIAN_POINT('',(-41.2927947172303,-1.3,10.5236110236165));
#26552=CARTESIAN_POINT('',(-24.9,-1.3,10.5236110236165));
#26553=CARTESIAN_POINT('Ctrl Pts',(-41.2927947172303,-1.3,10.5236110236165));
#26554=CARTESIAN_POINT('Ctrl Pts',(-40.8162222946067,-1.54189506348343,
10.7338267672599));
#26555=CARTESIAN_POINT('Ctrl Pts',(-40.3,-1.79511420941673,10.9538835567642));
#26556=CARTESIAN_POINT('Ctrl Pts',(-15.8,-1.79511420941674,10.9538835567642));
#26557=CARTESIAN_POINT('Ctrl Pts',(-15.9670634484609,-1.63121712795427,
10.8114509400566));
#26558=CARTESIAN_POINT('Ctrl Pts',(-16.1329130514351,-1.4659602821588,10.6678366379258));
#26559=CARTESIAN_POINT('Ctrl Pts',(-16.2963973586152,-1.3,10.5236110236165));
#26560=CARTESIAN_POINT('Origin',(-24.9,1.54755710470837,10.7387472901904));
#26561=CARTESIAN_POINT('',(-41.2927947172303,1.3,10.5236110236165));
#26562=CARTESIAN_POINT('Ctrl Pts',(-40.3,1.79511420941673,10.9538835567642));
#26563=CARTESIAN_POINT('Ctrl Pts',(-40.8162222946033,1.5418950634852,10.7338267672615));
#26564=CARTESIAN_POINT('Ctrl Pts',(-41.2927947172303,1.3,10.5236110236165));
#26565=CARTESIAN_POINT('',(-16.2963973586152,1.3,10.5236110236165));
#26566=CARTESIAN_POINT('',(-24.9,1.3,10.5236110236165));
#26567=CARTESIAN_POINT('Ctrl Pts',(-16.2963973586152,1.3,10.5236110236165));
#26568=CARTESIAN_POINT('Ctrl Pts',(-16.1329130514351,1.46596028215881,10.6678366379258));
#26569=CARTESIAN_POINT('Ctrl Pts',(-15.9670634484609,1.63121712795429,10.8114509400566));
#26570=CARTESIAN_POINT('Ctrl Pts',(-15.8,1.79511420941674,10.9538835567642));
#26571=CARTESIAN_POINT('Origin',(-16.05,0.,0.));
#26572=CARTESIAN_POINT('',(-16.3,1.3,10.519980988576));
#26573=CARTESIAN_POINT('Ctrl Pts',(-16.2963973586153,1.3,10.5236110236166));
#26574=CARTESIAN_POINT('Ctrl Pts',(-16.2981989900368,1.3,10.521795697712));
#26575=CARTESIAN_POINT('Ctrl Pts',(-16.3000000000001,1.3,10.519980988576));
#26576=CARTESIAN_POINT('',(-16.3,-1.3,10.519980988576));
#26577=CARTESIAN_POINT('Origin',(-16.3,0.,0.));
#26578=CARTESIAN_POINT('Ctrl Pts',(-16.3,-1.3,10.519980988576));
#26579=CARTESIAN_POINT('Ctrl Pts',(-16.2981989900368,-1.3,10.521795697712));
#26580=CARTESIAN_POINT('Ctrl Pts',(-16.2963973586152,-1.3,10.5236110236166));
#26581=CARTESIAN_POINT('Origin',(-16.3,0.,10.45));
#26582=CARTESIAN_POINT('',(-16.3,1.3,9.6));
#26583=CARTESIAN_POINT('',(-16.3,-1.3,11.3));
#26584=CARTESIAN_POINT('Origin',(-41.3,1.3,9.6));
#26585=CARTESIAN_POINT('',(-41.3,1.3,10.519980988576));
#26586=CARTESIAN_POINT('Ctrl Pts',(-41.3,1.3,10.519980988576));
#26587=CARTESIAN_POINT('Ctrl Pts',(-41.2963979800735,1.3,10.521795697712));
#26588=CARTESIAN_POINT('Ctrl Pts',(-41.2927947172303,1.3,10.5236110236165));
#26589=CARTESIAN_POINT('',(-41.3,1.3,4.8));
#26590=CARTESIAN_POINT('Origin',(-40.8,0.,0.));
#26591=CARTESIAN_POINT('',(-41.2927947172303,3.73947306290068,9.9223349161487));
#26592=CARTESIAN_POINT('Ctrl Pts',(-41.2927947172303,3.73947306290068,9.92233491614871));
#26593=CARTESIAN_POINT('Ctrl Pts',(-40.8162222946065,3.62297774856297,10.2208859542487));
#26594=CARTESIAN_POINT('Ctrl Pts',(-40.3,3.50102881923382,10.5334133692215));
#26595=CARTESIAN_POINT('',(-41.3,3.737786101502,9.9191206797487));
#26596=CARTESIAN_POINT('Ctrl Pts',(-41.2927947172303,3.73947306290068,9.92233491614871));
#26597=CARTESIAN_POINT('Ctrl Pts',(-41.2963979800734,3.73862943888804,9.92072752488803));
#26598=CARTESIAN_POINT('Ctrl Pts',(-41.3,3.737786101502,9.9191206797487));
#26599=CARTESIAN_POINT('Origin',(-41.3,0.,0.));
#26600=CARTESIAN_POINT('Origin',(-41.05,7.92498682077222,6.40017665706777));
#26601=CARTESIAN_POINT('',(-41.3,3.07788803224913,8.66178995710111));
#26602=CARTESIAN_POINT('',(-40.8,3.31024961827101,9.10451796992771));
#26603=CARTESIAN_POINT('',(-40.625,3.39157617337867,9.25947277441703));
#26604=CARTESIAN_POINT('',(-40.8,5.61243528496936,7.89623772261391));
#26605=CARTESIAN_POINT('',(-40.8,8.04116761378316,6.62154066348107));
#26606=CARTESIAN_POINT('',(-41.3,5.38007369894747,7.45350970978731));
#26607=CARTESIAN_POINT('',(-41.05,5.49625449195841,7.67487371620061));
#26608=CARTESIAN_POINT('',(-41.3,7.80880602776127,6.17881265065447));
#26609=CARTESIAN_POINT('Origin',(-41.3,3.31024961827101,9.10451796992771));
#26610=CARTESIAN_POINT('',(-16.3,3.31024961827101,9.10451796992771));
#26611=CARTESIAN_POINT('',(-41.3,3.31024961827101,9.10451796992771));
#26612=CARTESIAN_POINT('',(-16.3,5.61243528496936,7.89623772261391));
#26613=CARTESIAN_POINT('',(-16.3,3.31024961827101,9.10451796992771));
#26614=CARTESIAN_POINT('',(-41.3,5.61243528496936,7.89623772261391));
#26615=CARTESIAN_POINT('Origin',(-24.9,3.62025094106725,10.2278741426851));
#26616=CARTESIAN_POINT('',(-16.2963973586152,3.73947306290068,9.9223349161487));
#26617=CARTESIAN_POINT('',(-24.9,3.73947306290068,9.9223349161487));
#26618=CARTESIAN_POINT('Ctrl Pts',(-15.8,3.50102881923381,10.5334133692215));
#26619=CARTESIAN_POINT('Ctrl Pts',(-15.9670634484609,3.57996074016282,10.3311287789223));
#26620=CARTESIAN_POINT('Ctrl Pts',(-16.1329130514351,3.65954751601581,10.1271659441505));
#26621=CARTESIAN_POINT('Ctrl Pts',(-16.2963973586152,3.73947306290068,9.9223349161487));
#26622=CARTESIAN_POINT('Origin',(-24.9,6.36083846788017,8.78950284944721));
#26623=CARTESIAN_POINT('',(-41.2927947172303,6.04165872959903,8.7140546688349));
#26624=CARTESIAN_POINT('Ctrl Pts',(-40.3,6.6800182061613,8.86495103005952));
#26625=CARTESIAN_POINT('Ctrl Pts',(-40.8162222946031,6.35353829833807,8.78777722452791));
#26626=CARTESIAN_POINT('Ctrl Pts',(-41.2927947172303,6.04165872959903,8.7140546688349));
#26627=CARTESIAN_POINT('',(-16.2963973586152,6.04165872959903,8.7140546688349));
#26628=CARTESIAN_POINT('',(-24.9,6.04165872959903,8.7140546688349));
#26629=CARTESIAN_POINT('Ctrl Pts',(-16.2963973586152,6.04165872959903,8.7140546688349));
#26630=CARTESIAN_POINT('Ctrl Pts',(-16.1329130514352,6.25563424642728,8.76463451932043));
#26631=CARTESIAN_POINT('Ctrl Pts',(-15.9670634484612,6.46870281035421,8.81499998293205));
#26632=CARTESIAN_POINT('Ctrl Pts',(-15.8,6.68001820616131,8.86495103005952));
#26633=CARTESIAN_POINT('Origin',(-16.05,0.,0.));
#26634=CARTESIAN_POINT('',(-16.3,6.03997176820035,8.71084043243491));
#26635=CARTESIAN_POINT('Ctrl Pts',(-16.2963973586152,6.04165872959901,8.71405466883492));
#26636=CARTESIAN_POINT('Ctrl Pts',(-16.2981989900368,6.04081510558637,8.71244727757422));
#26637=CARTESIAN_POINT('Ctrl Pts',(-16.3000000000001,6.03997176820034,8.71084043243492));
#26638=CARTESIAN_POINT('',(-16.3,3.737786101502,9.91912067974871));
#26639=CARTESIAN_POINT('Origin',(-16.3,0.,0.));
#26640=CARTESIAN_POINT('Ctrl Pts',(-16.3,3.73778610150202,9.9191206797487));
#26641=CARTESIAN_POINT('Ctrl Pts',(-16.2981989900367,3.73862943888804,9.92072752488799));
#26642=CARTESIAN_POINT('Ctrl Pts',(-16.2963973586152,3.73947306290069,9.92233491614868));
#26643=CARTESIAN_POINT('Origin',(-16.3,4.85635714785739,9.25301546807604));
#26644=CARTESIAN_POINT('',(-16.3,5.61243528496936,7.89623772261391));
#26645=CARTESIAN_POINT('',(-16.3,4.10027901074542,10.6097932135382));
#26646=CARTESIAN_POINT('Origin',(-41.3,5.61243528496936,7.89623772261391));
#26647=CARTESIAN_POINT('',(-41.3,6.03997176820034,8.7108404324349));
#26648=CARTESIAN_POINT('Ctrl Pts',(-41.3,6.03997176820034,8.7108404324349));
#26649=CARTESIAN_POINT('Ctrl Pts',(-41.2963979800734,6.04081510558637,8.7124472775742));
#26650=CARTESIAN_POINT('Ctrl Pts',(-41.2927947172303,6.04165872959903,8.7140546688349));
#26651=CARTESIAN_POINT('',(-41.3,4.5263924803217,5.8269560440967));
#26652=CARTESIAN_POINT('Origin',(-40.8,0.,0.));
#26653=CARTESIAN_POINT('Origin',(-41.3,0.,0.));
#26654=CARTESIAN_POINT('Origin',(-41.05,0.,0.));
#26655=CARTESIAN_POINT('',(-41.3,4.71489017671731E-16,3.85));
#26656=CARTESIAN_POINT('Origin',(-41.3,0.,0.));
#26657=CARTESIAN_POINT('',(-40.8,-4.10256677714363E-16,3.35));
#26658=CARTESIAN_POINT('',(-41.05,4.40872847693047E-16,3.6));
#26659=CARTESIAN_POINT('Origin',(-40.8,0.,0.));
#26660=CARTESIAN_POINT('Origin',(-41.3,0.,0.));
#26661=CARTESIAN_POINT('',(-27.3,-4.10256677714363E-16,3.35));
#26662=CARTESIAN_POINT('',(-41.3,-4.10256677714363E-16,3.35));
#26663=CARTESIAN_POINT('Origin',(-27.3,0.,0.));
#26664=CARTESIAN_POINT('Origin',(-41.3,10.6,0.));
#26665=CARTESIAN_POINT('',(-41.3,2.61922150986056,7.78787391321573));
#26666=CARTESIAN_POINT('Origin',(-41.3,0.,0.));
#26667=CARTESIAN_POINT('Origin',(-41.3,0.,0.));
#26668=CARTESIAN_POINT('Origin',(-41.3,0.,0.));
#26669=CARTESIAN_POINT('Origin',(-41.3,0.,0.));
#26670=CARTESIAN_POINT('Origin',(-41.3,0.,0.));
#26671=CARTESIAN_POINT('Origin',(-41.3,0.,0.));
#26672=CARTESIAN_POINT('Origin',(-41.3,0.,0.));
#26673=CARTESIAN_POINT('Origin',(-41.3,0.,0.));
#26674=CARTESIAN_POINT('Origin',(-41.3,0.,0.));
#26675=CARTESIAN_POINT('',(-41.3,-1.3,10.519980988576));
#26676=CARTESIAN_POINT('Origin',(-41.3,0.,0.));
#26677=CARTESIAN_POINT('',(-41.3,-1.3,5.65));
#26678=CARTESIAN_POINT('Origin',(-27.3,0.,0.));
#26679=CARTESIAN_POINT('Origin',(75.,-3.,12.5));
#26680=CARTESIAN_POINT('',(75.,-3.,12.1346610995116));
#26681=CARTESIAN_POINT('',(75.,3.,12.1346610995116));
#26682=CARTESIAN_POINT('Origin',(75.,0.,0.));
#26683=CARTESIAN_POINT('',(75.,-3.,9.));
#26684=CARTESIAN_POINT('',(75.,-3.,12.5));
#26685=CARTESIAN_POINT('',(75.,3.,9.));
#26686=CARTESIAN_POINT('',(75.,3.,9.));
#26687=CARTESIAN_POINT('',(75.,3.,12.5));
#26688=CARTESIAN_POINT('Origin',(75.,3.,12.5));
#26689=CARTESIAN_POINT('',(115.,3.,12.1346610995116));
#26690=CARTESIAN_POINT('',(109.05,3.,12.1346610995116));
#26691=CARTESIAN_POINT('',(115.,3.,9.));
#26692=CARTESIAN_POINT('',(115.,3.,9.));
#26693=CARTESIAN_POINT('',(115.,3.,12.5));
#26694=CARTESIAN_POINT('Origin',(115.,-3.,12.5));
#26695=CARTESIAN_POINT('',(115.,-3.,12.1346610995116));
#26696=CARTESIAN_POINT('',(109.05,-3.,12.1346610995116));
#26697=CARTESIAN_POINT('',(115.,-3.,9.));
#26698=CARTESIAN_POINT('',(115.,-3.,12.5));
#26699=CARTESIAN_POINT('',(75.,-3.,9.));
#26700=CARTESIAN_POINT('Origin',(115.,3.,12.5));
#26701=CARTESIAN_POINT('Origin',(115.,0.,0.));
#26702=CARTESIAN_POINT('',(115.,-3.,9.));
#26703=CARTESIAN_POINT('Origin',(95.,0.,9.));
#26704=CARTESIAN_POINT('Origin',(-41.3,4.10027901074542,10.6097932135382));
#26705=CARTESIAN_POINT('Origin',(-40.8,0.,0.));
#26706=CARTESIAN_POINT('Origin',(-40.8,0.,0.));
#26707=CARTESIAN_POINT('Origin',(-40.8,0.,0.));
#26708=CARTESIAN_POINT('Origin',(-40.8,0.,0.));
#26709=CARTESIAN_POINT('Origin',(-16.3,2.50084869180498,-10.1463419921022));
#26710=CARTESIAN_POINT('Origin',(-40.8,0.,0.));
#26711=CARTESIAN_POINT('Origin',(-40.8,0.,0.));
#26712=CARTESIAN_POINT('Origin',(-40.8,0.,0.));
#26713=CARTESIAN_POINT('Origin',(-40.8,0.,0.));
#26714=CARTESIAN_POINT('Origin',(-40.8,0.,0.));
#26715=CARTESIAN_POINT('Origin',(-41.3,-1.3,11.3));
#26716=CARTESIAN_POINT('Ctrl Pts',(-41.2927947172303,-1.3,10.5236110236165));
#26717=CARTESIAN_POINT('Ctrl Pts',(-41.2963979800735,-1.3,10.521795697712));
#26718=CARTESIAN_POINT('Ctrl Pts',(-41.3,-1.3,10.519980988576));
#26719=CARTESIAN_POINT('Origin',(-40.8,0.,0.));
#26720=CARTESIAN_POINT('Origin',(-9.5,15.,0.));
#26721=CARTESIAN_POINT('',(-9.49999999999999,-15.,-1.83697019872103E-15));
#26722=CARTESIAN_POINT('Origin',(-9.49999999999999,0.,0.));
#26723=CARTESIAN_POINT('Origin',(2.25,0.,0.));
#26724=CARTESIAN_POINT('',(14.,-15.,-1.83697019872103E-15));
#26725=CARTESIAN_POINT('Origin',(14.,0.,0.));
#26726=CARTESIAN_POINT('',(2.25,-15.,-1.83697019872103E-15));
#26727=CARTESIAN_POINT('Origin',(14.,14.,0.));
#26728=CARTESIAN_POINT('',(14.,-14.,-1.71450551880629E-15));
#26729=CARTESIAN_POINT('Origin',(14.,0.,0.));
#26730=CARTESIAN_POINT('Origin',(39.9,0.,0.));
#26731=CARTESIAN_POINT('',(65.8,-14.,-1.71450551880629E-15));
#26732=CARTESIAN_POINT('Origin',(65.8,0.,0.));
#26733=CARTESIAN_POINT('',(39.9,-14.,-1.71450551880629E-15));
#26734=CARTESIAN_POINT('Origin',(65.8,12.5,0.));
#26735=CARTESIAN_POINT('',(65.8,-12.5,-1.53080849893419E-15));
#26736=CARTESIAN_POINT('Origin',(65.8,0.,0.));
#26737=CARTESIAN_POINT('Origin',(109.05,0.,0.));
#26738=CARTESIAN_POINT('',(152.3,-12.5,-1.53080849893419E-15));
#26739=CARTESIAN_POINT('Origin',(152.3,0.,0.));
#26740=CARTESIAN_POINT('',(109.05,-12.5,-1.53080849893419E-15));
#26741=CARTESIAN_POINT('Origin',(152.55,0.,0.));
#26742=CARTESIAN_POINT('',(152.8,-12.,-1.46957615897682E-15));
#26743=CARTESIAN_POINT('Origin',(152.8,0.,0.));
#26744=CARTESIAN_POINT('',(152.55,-12.25,-1.50019232895551E-15));
#26745=CARTESIAN_POINT('Origin',(152.8,0.,0.));
#38480=UNCERTAINTY_MEASURE_WITH_UNIT(LENGTH_MEASURE(0.01),#38508,
'DISTANCE_ACCURACY_VALUE',
'Maximum model space distance between geometric entities at asserted c
onnectivities');
#38490=UNCERTAINTY_MEASURE_WITH_UNIT(LENGTH_MEASURE(0.01),#38508,
'DISTANCE_ACCURACY_VALUE',
'Maximum model space distance between geometric entities at asserted c
onnectivities');
#38497=(
GEOMETRIC_REPRESENTATION_CONTEXT(3)
GLOBAL_UNCERTAINTY_ASSIGNED_CONTEXT((#38480))
GLOBAL_UNIT_ASSIGNED_CONTEXT((#38508,#38510,#38511))
REPRESENTATION_CONTEXT('','3D')
);
#38507=(
GEOMETRIC_REPRESENTATION_CONTEXT(3)
GLOBAL_UNCERTAINTY_ASSIGNED_CONTEXT((#38490))
GLOBAL_UNIT_ASSIGNED_CONTEXT((#38508,#38510,#38511))
REPRESENTATION_CONTEXT('','3D')
);
#38508=(
LENGTH_UNIT()
NAMED_UNIT(*)
SI_UNIT(.MILLI.,.METRE.)
);
#38510=(
NAMED_UNIT(*)
PLANE_ANGLE_UNIT()
SI_UNIT($,.RADIAN.)
);
#38511=(
NAMED_UNIT(*)
SI_UNIT($,.STERADIAN.)
SOLID_ANGLE_UNIT()
);
#38518=SHAPE_DEFINITION_REPRESENTATION(#38534,#38580);
#38534=PRODUCT_DEFINITION_SHAPE('',$,#38597);
#38580=SHAPE_REPRESENTATION('',(#15950),#38497);
#38590=PRODUCT_DEFINITION_CONTEXT('part definition',#38640,'design');
#38597=PRODUCT_DEFINITION('2026-10-26-01-10-51-970',
'09_Drive_Shaft_SAE_B_13T',#38613,#38590);
#38613=PRODUCT_DEFINITION_FORMATION('',$,#38648);
#38640=APPLICATION_CONTEXT(
'Core Data for Automotive Mechanical Design Process');
#38641=PRODUCT_CONTEXT('part definition',#38640,'mechanical');
#38648=PRODUCT('2026-10-26-01-10-51-970','09_Drive_Shaft_SAE_B_13T',$,(#38641));
#38714=COLOUR_RGB('Grey',0.48,0.52,0.57);
#38715=FILL_AREA_STYLE_COLOUR('',#38714);
#38716=FILL_AREA_STYLE('',(#38715));
#38717=SURFACE_STYLE_FILL_AREA(#38716);
#38718=SURFACE_SIDE_STYLE('',(#38717));
#38719=SURFACE_STYLE_USAGE(.BOTH.,#38718);
#38720=PRESENTATION_STYLE_ASSIGNMENT((#38719));
ENDSEC;
END-ISO-10303-21;
